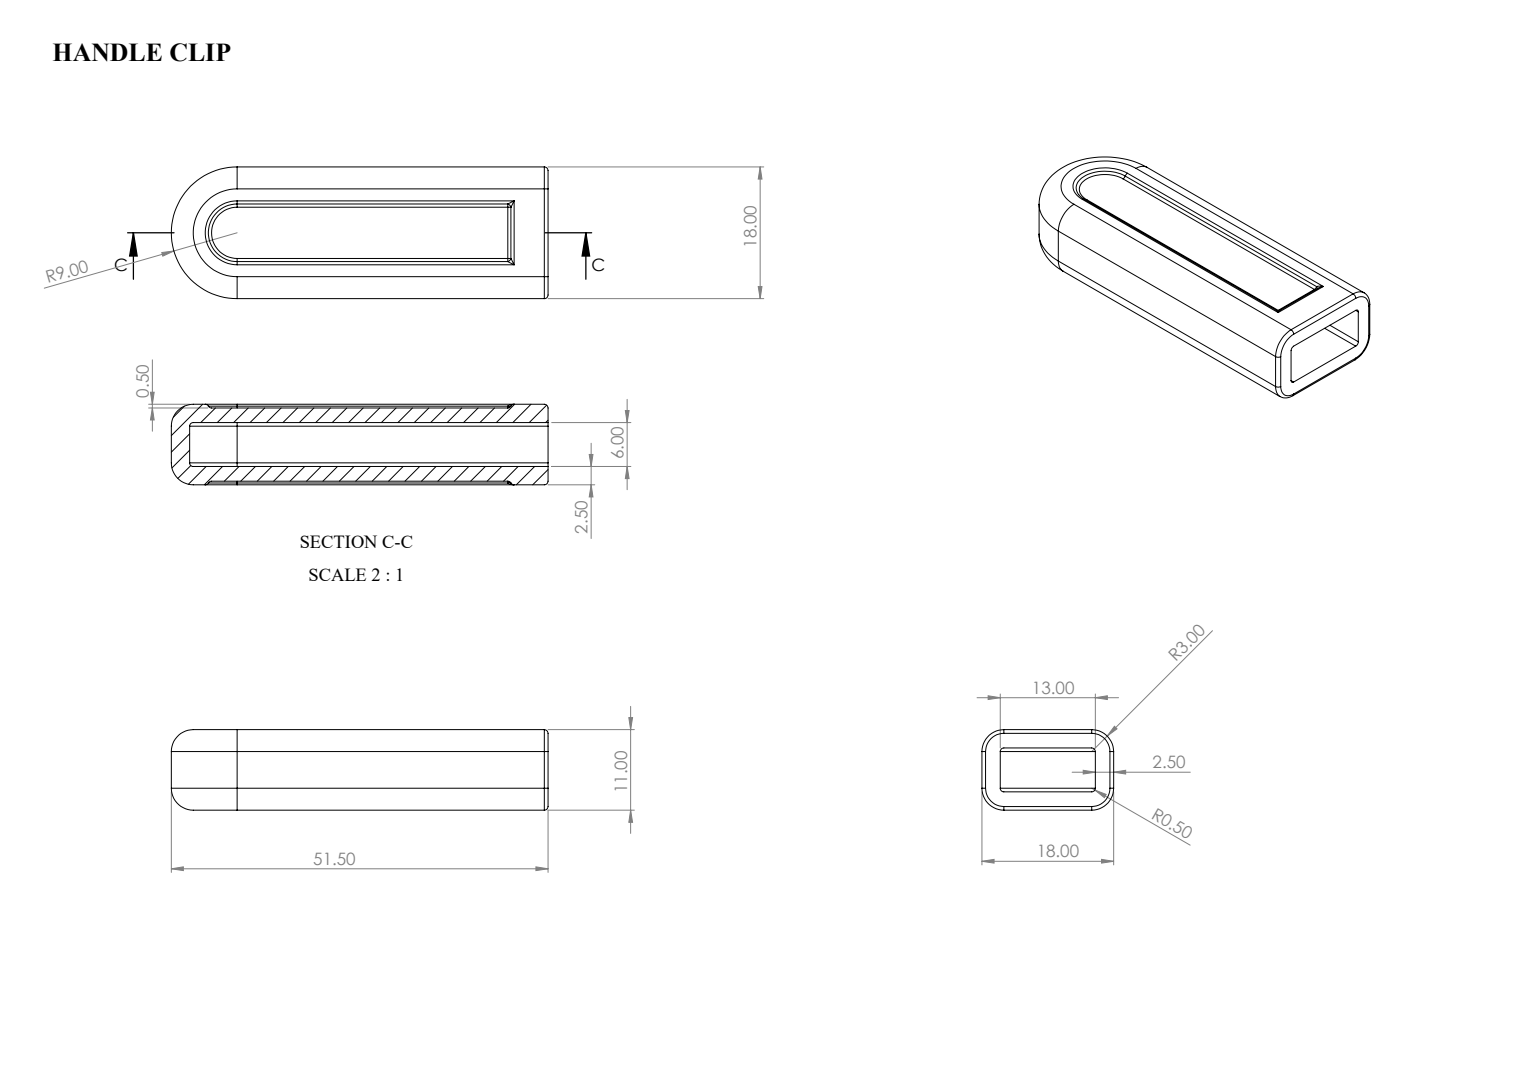
ISO-10303-21;
HEADER;
FILE_DESCRIPTION (('STEP AP214'),
    '1' );
FILE_NAME ('Handle Clip.step',
    '2026-10-06T08:09:25',
    ( '' ),
    ( '' ),
    'SwSTEP 2.0',
    'SolidWorks 2021',
    '' );
FILE_SCHEMA (( 'AUTOMOTIVE_DESIGN' ));
ENDSEC;

DATA;
#11=DIRECTION ( 'NONE',  ( 1.000000000000000000, -4.190823558986610327E-31, 1.733449886265890494E-32 ) ) ;
#13=CARTESIAN_POINT ( 'NONE',  ( 2.775557561562891351E-14, 10.75000000000000000, -10.43301270189220276 ) ) ;
#17=CARTESIAN_POINT ( 'NONE',  ( 2.775557561562891351E-14, 11.00000000000000000, -6.499999999999950262 ) ) ;
#23=CARTESIAN_POINT ( 'NONE',  ( 2.775557561562891351E-14, 8.000000000000003553, -6.499999999999950262 ) ) ;
#34=ORIENTED_EDGE ( 'NONE', *, *, #10798, .T. ) ;
#55=EDGE_CURVE ( 'NONE', #3237, #11583, #13792, .T. ) ;
#60=ORIENTED_EDGE ( 'NONE', *, *, #16971, .F. ) ;
#90=CIRCLE ( 'NONE', #20736, 0.5000000000000004441 ) ;
#104=CARTESIAN_POINT ( 'NONE',  ( 37.00000000000030553, 10.74999999999998579, -10.43301270189227559 ) ) ;
#180=VERTEX_POINT ( 'NONE', #3214 ) ;
#181=ORIENTED_EDGE ( 'NONE', *, *, #18463, .F. ) ;
#221=CARTESIAN_POINT ( 'NONE',  ( 37.36637401601599606, 0.3137297356303613283, -10.36637401601559105 ) ) ;
#222=ADVANCED_FACE ( 'NONE', ( #21089 ), #12579, .F. ) ;
#254=CARTESIAN_POINT ( 'NONE',  ( 37.09721192197999073, 0.1772999597157984553, -2.518381337117822305 ) ) ;
#264=DIRECTION ( 'NONE',  ( 1.000000000000000000, -4.190823558986610327E-31, 1.733449886265890494E-32 ) ) ;
#279=CIRCLE ( 'NONE', #13429, 0.5000000000000022204 ) ;
#288=LINE ( 'NONE', #14177, #16241 ) ;
#290=VECTOR ( 'NONE', #21577, 1000.000000000000000 ) ;
#337=ADVANCED_FACE ( 'NONE', ( #3665 ), #4392, .F. ) ;
#370=EDGE_CURVE ( 'NONE', #12160, #6309, #12209, .T. ) ;
#393=EDGE_CURVE ( 'NONE', #22556, #13205, #17081, .T. ) ;
#423=EDGE_LOOP ( 'NONE', ( #4977, #10308, #16171, #6608 ) ) ;
#435=DIRECTION ( 'NONE',  ( -1.000000000000000000, 4.190823558986610327E-31, -1.733449886265890494E-32 ) ) ;
#444=VECTOR ( 'NONE', #613, 1000.000000000000000 ) ;
#448=EDGE_CURVE ( 'NONE', #12541, #7709, #4224, .T. ) ;
#452=CARTESIAN_POINT ( 'NONE',  ( 37.00000000000006395, 10.75000000000000000, -10.43301270189220276 ) ) ;
#471=CARTESIAN_POINT ( 'NONE',  ( 42.50000000000014921, 2.999999999999999112, -14.99999999999998579 ) ) ;
#473=ADVANCED_FACE ( 'NONE', ( #13534 ), #11758, .F. ) ;
#478=AXIS2_PLACEMENT_3D ( 'NONE', #12426, #1725, #23034 ) ;
#481=ORIENTED_EDGE ( 'NONE', *, *, #4021, .F. ) ;
#485=PLANE ( 'NONE',  #3877 ) ;
#513=ORIENTED_EDGE ( 'NONE', *, *, #17633, .T. ) ;
#518=ORIENTED_EDGE ( 'NONE', *, *, #5953, .T. ) ;
#534=DIRECTION ( 'NONE',  ( 1.000000000000000000, -4.190823558986610327E-31, 1.733449886265890494E-32 ) ) ;
#539=CARTESIAN_POINT ( 'NONE',  ( 37.46001462128848658, 10.83019807384524391, -2.539985378711986819 ) ) ;
#567=EDGE_CURVE ( 'NONE', #9447, #4397, #14113, .T. ) ;
#591=EDGE_CURVE ( 'NONE', #7197, #2718, #10576, .T. ) ;
#594=EDGE_CURVE ( 'NONE', #12892, #3237, #956, .T. ) ;
#599=EDGE_LOOP ( 'NONE', ( #7573, #20564, #19035, #15482 ) ) ;
#602=CARTESIAN_POINT ( 'NONE',  ( 37.35148779274769026, 0.3618892054749011655, -2.648512207251555228 ) ) ;
#613=DIRECTION ( 'NONE',  ( 1.000000000000000000, -4.437342591868175641E-31, 3.330669073875457788E-16 ) ) ;
#614=DIRECTION ( 'NONE',  ( 0.000000000000000000, 0.000000000000000000, 1.000000000000000000 ) ) ;
#621=FACE_OUTER_BOUND ( 'NONE', #4835, .T. ) ;
#633=ORIENTED_EDGE ( 'NONE', *, *, #21096, .F. ) ;
#637=DIRECTION ( 'NONE',  ( 3.330669073875457788E-16, 0.000000000000000000, -1.000000000000000000 ) ) ;
#640=DIRECTION ( 'NONE',  ( -0.000000000000000000, 1.000000000000000000, 4.190823558986611203E-31 ) ) ;
#643=EDGE_CURVE ( 'NONE', #2718, #1098, #1705, .T. ) ;
#649=CARTESIAN_POINT ( 'NONE',  ( 2.775557561562891351E-14, 8.499999999999984013, -0.4999999999999865663 ) ) ;
#663=ORIENTED_EDGE ( 'NONE', *, *, #7766, .F. ) ;
#698=CARTESIAN_POINT ( 'NONE',  ( 2.775557561562891351E-14, 8.499999999999984013, -0.4999999999999865663 ) ) ;
#732=CARTESIAN_POINT ( 'NONE',  ( 2.775557561562891351E-14, 2.999999999999992450, -0.4999999999999865663 ) ) ;
#842=AXIS2_PLACEMENT_3D ( 'NONE', #19098, #1117, #4968 ) ;
#862=ORIENTED_EDGE ( 'NONE', *, *, #5242, .F. ) ;
#863=TOROIDAL_SURFACE ( 'NONE', #8360, 4.366025403784441039, 0.5000000000000000000 ) ;
#871=CARTESIAN_POINT ( 'NONE',  ( 37.43301270189236618, 10.75000000000000000, -2.999999999999988898 ) ) ;
#872=AXIS2_PLACEMENT_3D ( 'NONE', #21088, #8383, #18976 ) ;
#892=ORIENTED_EDGE ( 'NONE', *, *, #22327, .T. ) ;
#895=ORIENTED_EDGE ( 'NONE', *, *, #16706, .T. ) ;
#896=EDGE_CURVE ( 'NONE', #16369, #9334, #7402, .T. ) ;
#905=DIRECTION ( 'NONE',  ( 4.190823558986625216E-31, -1.000000000000000000, 4.190823558986625216E-31 ) ) ;
#906=VECTOR ( 'NONE', #1561, 1000.000000000000000 ) ;
#909=CIRCLE ( 'NONE', #17036, 0.5000000000000022204 ) ;
#918=CARTESIAN_POINT ( 'NONE',  ( 37.57823792062865209, 0.08880391167987312928, -10.29045043747235333 ) ) ;
#956=CIRCLE ( 'NONE', #20106, 3.933012701892234730 ) ;
#966=FACE_OUTER_BOUND ( 'NONE', #6498, .T. ) ;
#971=DIRECTION ( 'NONE',  ( 0.000000000000000000, 0.000000000000000000, 1.000000000000000000 ) ) ;
#977=ORIENTED_EDGE ( 'NONE', *, *, #23196, .F. ) ;
#980=ORIENTED_EDGE ( 'NONE', *, *, #4067, .T. ) ;
#999=CARTESIAN_POINT ( 'NONE',  ( 37.00000000000011369, 10.49999999999999822, -10.00000000000000888 ) ) ;
#1005=ORIENTED_EDGE ( 'NONE', *, *, #896, .T. ) ;
#1019=FACE_OUTER_BOUND ( 'NONE', #2701, .T. ) ;
#1038=ORIENTED_EDGE ( 'NONE', *, *, #6940, .T. ) ;
#1043=DIRECTION ( 'NONE',  ( -4.190823558986626092E-31, 1.000000000000000000, 4.190823558986610327E-31 ) ) ;
#1069=ADVANCED_FACE ( 'NONE', ( #22690 ), #22337, .T. ) ;
#1071=EDGE_CURVE ( 'NONE', #22556, #2883, #22565, .T. ) ;
#1076=CARTESIAN_POINT ( 'NONE',  ( 37.00000000000011369, 11.00000000000000000, -6.499999999999950262 ) ) ;
#1098=VERTEX_POINT ( 'NONE', #13743 ) ;
#1117=DIRECTION ( 'NONE',  ( -1.000000000000000000, 4.190823558986610327E-31, -1.733449886265890494E-32 ) ) ;
#1149=SHAPE_REPRESENTATION_RELATIONSHIP ( 'NONE' , 'NONE' ,  #1164, #3571 ) ;
#1154=ORIENTED_EDGE ( 'NONE', *, *, #9823, .F. ) ;
#1164=SHAPE_REPRESENTATION ( 'Handle Clip', ( #22115 ), #13848 ) ;
#1185=CARTESIAN_POINT ( 'NONE',  ( 2.775557561562891351E-14, 0.5000000000000004441, -3.000000000000002665 ) ) ;
#1188=SPHERICAL_SURFACE ( 'NONE', #17017, 0.5000000000000000000 ) ;
#1193=CARTESIAN_POINT ( 'NONE',  ( 37.43301270189239460, 0.2500000000000002220, -9.999999999999953815 ) ) ;
#1228=CIRCLE ( 'NONE', #14361, 0.5000000000000004441 ) ;
#1229=DIRECTION ( 'NONE',  ( -0.000000000000000000, 1.000000000000000000, 4.190823558986611203E-31 ) ) ;
#1236=ORIENTED_EDGE ( 'NONE', *, *, #23063, .T. ) ;
#1238=ORIENTED_EDGE ( 'NONE', *, *, #15588, .F. ) ;
#1256=AXIS2_PLACEMENT_3D ( 'NONE', #7873, #3869, #9180 ) ;
#1287=CYLINDRICAL_SURFACE ( 'NONE', #4701, 0.5000000000000017764 ) ;
#1302=DIRECTION ( 'NONE',  ( -4.190823558986625216E-31, 1.000000000000000000, -4.190823558986625216E-31 ) ) ;
#1322=ORIENTED_EDGE ( 'NONE', *, *, #5382, .T. ) ;
#1341=CARTESIAN_POINT ( 'NONE',  ( 37.00000000000017053, 0.2500000000000002220, -10.43301270189217433 ) ) ;
#1361=AXIS2_PLACEMENT_3D ( 'NONE', #12480, #2122, #5209 ) ;
#1365=DIRECTION ( 'NONE',  ( -1.000000000000000000, 4.190823558986610327E-31, -1.733449886265890494E-32 ) ) ;
#1366=STYLED_ITEM ( 'NONE', ( #22113 ), #21090 ) ;
#1373=DIRECTION ( 'NONE',  ( 0.000000000000000000, 9.769962616701412266E-15, 1.000000000000000000 ) ) ;
#1379=FILL_AREA_STYLE ('',( #17353 ) ) ;
#1390=CARTESIAN_POINT ( 'NONE',  ( 42.00000000000020606, 0.4999999999999865663, -0.4999999999999449329 ) ) ;
#1394=DIRECTION ( 'NONE',  ( 3.330669073875454830E-16, 0.000000000000000000, -1.000000000000000000 ) ) ;
#1416=CARTESIAN_POINT ( 'NONE',  ( 2.775557561562891351E-14, 11.00000000000000000, -9.999999999999968026 ) ) ;
#1455=EDGE_CURVE ( 'NONE', #5339, #2694, #13565, .T. ) ;
#1462=CIRCLE ( 'NONE', #22131, 4.366025403784456138 ) ;
#1467=EDGE_CURVE ( 'NONE', #15040, #9447, #5099, .T. ) ;
#1476=DIRECTION ( 'NONE',  ( 0.000000000000000000, 0.000000000000000000, -1.000000000000000000 ) ) ;
#1479=DIRECTION ( 'NONE',  ( -1.000000000000000000, 0.000000000000000000, 0.000000000000000000 ) ) ;
#1481=DIRECTION ( 'NONE',  ( 0.000000000000000000, -4.190823558986610327E-31, 1.000000000000000000 ) ) ;
#1526=FACE_OUTER_BOUND ( 'NONE', #8749, .T. ) ;
#1536=CARTESIAN_POINT ( 'NONE',  ( 37.18301270189237329, 10.90849364905388619, -2.475480947161653233 ) ) ;
#1556=DIRECTION ( 'NONE',  ( 0.000000000000000000, 0.000000000000000000, 1.000000000000000000 ) ) ;
#1559=DIRECTION ( 'NONE',  ( -4.190823558986625216E-31, 1.000000000000000000, -4.190823558986625216E-31 ) ) ;
#1561=DIRECTION ( 'NONE',  ( -4.190823558986625216E-31, 1.000000000000000000, -4.190823558986625216E-31 ) ) ;
#1562=CYLINDRICAL_SURFACE ( 'NONE', #18135, 0.5000000000000022204 ) ;
#1581=ORIENTED_EDGE ( 'NONE', *, *, #20471, .T. ) ;
#1582=CARTESIAN_POINT ( 'NONE',  ( 42.00000000000012079, 2.999999999999999112, -12.49999999999999645 ) ) ;
#1591=ADVANCED_FACE ( 'NONE', ( #21452 ), #10724, .T. ) ;
#1605=ADVANCED_FACE ( 'NONE', ( #9075 ), #23102, .F. ) ;
#1624=CARTESIAN_POINT ( 'NONE',  ( 37.73505106183036162, 10.99999999999229061, -10.73505106183359104 ) ) ;
#1630=LINE ( 'NONE', #8813, #3292 ) ;
#1646=DIRECTION ( 'NONE',  ( 4.190823558986625216E-31, -1.000000000000000000, 4.190823558986625216E-31 ) ) ;
#1656=DIRECTION ( 'NONE',  ( -1.000000000000000000, 4.190823558986610327E-31, -1.733449886265890494E-32 ) ) ;
#1658=CARTESIAN_POINT ( 'NONE',  ( 37.68301270189240171, 11.00000000000000533, -2.499999999999975575 ) ) ;
#1669=VERTEX_POINT ( 'NONE', #11524 ) ;
#1705=CIRCLE ( 'NONE', #16346, 2.500000000000009326 ) ;
#1725=DIRECTION ( 'NONE',  ( 4.392831559381931789E-32, 2.168404344970994323E-16, 1.000000000000000000 ) ) ;
#1727=FACE_OUTER_BOUND ( 'NONE', #17848, .T. ) ;
#1734=CARTESIAN_POINT ( 'NONE',  ( 37.77870956205628516, 11.00000000000000000, -10.69139372032722335 ) ) ;
#1746=ORIENTED_EDGE ( 'NONE', *, *, #17889, .F. ) ;
#1759=CARTESIAN_POINT ( 'NONE',  ( 2.775557561562891351E-14, 8.500000000000003553, -6.499999999999950262 ) ) ;
#1764=DIRECTION ( 'NONE',  ( 1.000000000000000000, -4.190823558986610327E-31, 1.733449886265890494E-32 ) ) ;
#1823=CARTESIAN_POINT ( 'NONE',  ( 2.775557561562891351E-14, 11.00000000000000000, -12.50000000000001066 ) ) ;
#1836=CARTESIAN_POINT ( 'NONE',  ( 42.50000000000014921, 5.500000000000001776, 2.000000000000071054 ) ) ;
#1890=DIRECTION ( 'NONE',  ( -1.000000000000000000, 4.190823558986610327E-31, -1.733449886265890494E-32 ) ) ;
#1926=CIRCLE ( 'NONE', #17697, 3.000000000000011546 ) ;
#1960=CARTESIAN_POINT ( 'NONE',  ( 37.45482484129320966, 0.2122202663360098496, -10.04362427881557274 ) ) ;
#1965=EDGE_LOOP ( 'NONE', ( #1982, #10746, #15822, #4725 ) ) ;
#1966=EDGE_CURVE ( 'NONE', #3408, #6309, #5169, .T. ) ;
#1982=ORIENTED_EDGE ( 'NONE', *, *, #448, .F. ) ;
#1985=LINE ( 'NONE', #7524, #10565 ) ;
#2000=ORIENTED_EDGE ( 'NONE', *, *, #370, .T. ) ;
#2003=ORIENTED_EDGE ( 'NONE', *, *, #17889, .T. ) ;
#2006=EDGE_CURVE ( 'NONE', #13205, #15190, #3678, .T. ) ;
#2009=CIRCLE ( 'NONE', #18541, 3.933012701892234730 ) ;
#2016=CARTESIAN_POINT ( 'NONE',  ( 2.775557561562891351E-14, 10.49999999999999822, -9.999999999999968026 ) ) ;
#2020=CARTESIAN_POINT ( 'NONE',  ( 42.50000000000020606, 2.499999999999998668, -13.00000000000002487 ) ) ;
#2030=ORIENTED_EDGE ( 'NONE', *, *, #21313, .F. ) ;
#2045=DIRECTION ( 'NONE',  ( -1.000000000000000000, 4.437342591868175641E-31, -3.330669073875457788E-16 ) ) ;
#2108=DIRECTION ( 'NONE',  ( 1.000000000000000000, -4.190823558986610327E-31, 1.733449886265890494E-32 ) ) ;
#2112=SHAPE_DEFINITION_REPRESENTATION ( #15484, #1164 ) ;
#2117=ORIENTED_EDGE ( 'NONE', *, *, #5918, .F. ) ;
#2122=DIRECTION ( 'NONE',  ( 1.733449886265891589E-32, -4.190823558986610327E-31, 1.000000000000000000 ) ) ;
#2130=LINE ( 'NONE', #16478, #444 ) ;
#2141=AXIS2_PLACEMENT_3D ( 'NONE', #5036, #12437, #3627 ) ;
#2143=ORIENTED_EDGE ( 'NONE', *, *, #22541, .T. ) ;
#2148=CIRCLE ( 'NONE', #6298, 0.5000000000000012212 ) ;
#2162=DIRECTION ( 'NONE',  ( 0.000000000000000000, 0.000000000000000000, -1.000000000000000000 ) ) ;
#2181=ORIENTED_EDGE ( 'NONE', *, *, #14586, .T. ) ;
#2182=AXIS2_PLACEMENT_3D ( 'NONE', #11996, #13664, #17057 ) ;
#2187=CARTESIAN_POINT ( 'NONE',  ( 2.775557561562891351E-14, 2.999999999999999112, -12.50000000000001066 ) ) ;
#2193=CARTESIAN_POINT ( 'NONE',  ( 5.551115123125782702E-14, 3.000000000000027089, 2.500000000000071498 ) ) ;
#2247=ORIENTED_EDGE ( 'NONE', *, *, #14877, .T. ) ;
#2355=CARTESIAN_POINT ( 'NONE',  ( 37.29045043747246524, 0.08880391167994924895, -2.421762079371568621 ) ) ;
#2357=VERTEX_POINT ( 'NONE', #12661 ) ;
#2365=CARTESIAN_POINT ( 'NONE',  ( 42.00000000000014921, 10.49999999999999822, -12.50000000000005329 ) ) ;
#2406=CIRCLE ( 'NONE', #14045, 6.500000000000023981 ) ;
#2436=AXIS2_PLACEMENT_3D ( 'NONE', #5086, #19320, #17907 ) ;
#2449=VECTOR ( 'NONE', #22347, 1000.000000000000000 ) ;
#2453=CARTESIAN_POINT ( 'NONE',  ( 42.00000000000020606, -1.387778780781445676E-14, -0.4999999999999449329 ) ) ;
#2463=EDGE_CURVE ( 'NONE', #3085, #7197, #14612, .T. ) ;
#2469=LINE ( 'NONE', #6127, #2740 ) ;
#2524=ORIENTED_EDGE ( 'NONE', *, *, #1467, .T. ) ;
#2536=LINE ( 'NONE', #7952, #7258 ) ;
#2541=VECTOR ( 'NONE', #5687, 1000.000000000000000 ) ;
#2546=CARTESIAN_POINT ( 'NONE',  ( 37.73505106183116453, 7.752354164078167471E-12, -10.73505106183309543 ) ) ;
#2547=VECTOR ( 'NONE', #4832, 1000.000000000000000 ) ;
#2570=DIRECTION ( 'NONE',  ( 1.000000000000000000, -4.190823558986610327E-31, 1.733449886265890494E-32 ) ) ;
#2575=DIRECTION ( 'NONE',  ( 4.190823558986625216E-31, -1.000000000000000000, 4.190823558986625216E-31 ) ) ;
#2586=CARTESIAN_POINT ( 'NONE',  ( 2.775557561562891351E-14, 2.499999999999998668, -6.499999999999950262 ) ) ;
#2589=ORIENTED_EDGE ( 'NONE', *, *, #13484, .F. ) ;
#2615=( BOUNDED_CURVE ( )  B_SPLINE_CURVE ( 3, ( #11377, #12923, #10910, #452 ),
 .UNSPECIFIED., .F., .F. ) 
 B_SPLINE_CURVE_WITH_KNOTS ( ( 4, 4 ),
 ( 1.570796326794896558, 2.617993877991555252 ),
 .UNSPECIFIED. ) 
 CURVE ( )  GEOMETRIC_REPRESENTATION_ITEM ( )  RATIONAL_B_SPLINE_CURVE ( ( 1.000000000000000000, 0.9106836025229487763, 0.9106836025229487763, 1.000000000000000000 ) ) 
 REPRESENTATION_ITEM ( '' )  );
#2625=AXIS2_PLACEMENT_3D ( 'NONE', #11795, #8154, #20750 ) ;
#2631=CARTESIAN_POINT ( 'NONE',  ( 42.00000000000014921, 2.999999999999999112, -15.00000000000001421 ) ) ;
#2656=AXIS2_PLACEMENT_3D ( 'NONE', #6369, #13310, #14944 ) ;
#2681=CARTESIAN_POINT ( 'NONE',  ( 2.775557561562891351E-14, 8.500000000000003553, -6.499999999999950262 ) ) ;
#2693=ORIENTED_EDGE ( 'NONE', *, *, #12821, .F. ) ;
#2694=VERTEX_POINT ( 'NONE', #20789 ) ;
#2696=CIRCLE ( 'NONE', #9847, 0.5000000000000004441 ) ;
#2701=EDGE_LOOP ( 'NONE', ( #12986, #7252, #2247, #12420 ) ) ;
#2708=CYLINDRICAL_SURFACE ( 'NONE', #11715, 9.000000000000031974 ) ;
#2714=DIRECTION ( 'NONE',  ( 0.000000000000000000, 0.000000000000000000, 1.000000000000000000 ) ) ;
#2718=VERTEX_POINT ( 'NONE', #22660 ) ;
#2722=ORIENTED_EDGE ( 'NONE', *, *, #7766, .T. ) ;
#2740=VECTOR ( 'NONE', #16468, 1000.000000000000000 ) ;
#2758=AXIS2_PLACEMENT_3D ( 'NONE', #16955, #13884, #15520 ) ;
#2805=DIRECTION ( 'NONE',  ( -4.190823558986626092E-31, 1.000000000000000000, 4.190823558986610327E-31 ) ) ;
#2807=( BOUNDED_CURVE ( )  B_SPLINE_CURVE ( 3, ( #5658, #9761, #18585, #18238 ),
 .UNSPECIFIED., .F., .T. ) 
 B_SPLINE_CURVE_WITH_KNOTS ( ( 4, 4 ),
 ( 3.665191429188058070, 4.712388980384689674 ),
 .UNSPECIFIED. ) 
 CURVE ( )  GEOMETRIC_REPRESENTATION_ITEM ( )  RATIONAL_B_SPLINE_CURVE ( ( 1.000000000000000000, 0.9106836025229534393, 0.9106836025229534393, 1.000000000000000000 ) ) 
 REPRESENTATION_ITEM ( '' )  );
#2841=FACE_OUTER_BOUND ( 'NONE', #18394, .T. ) ;
#2843=CARTESIAN_POINT ( 'NONE',  ( 2.775557561562891351E-14, 2.499999999999998668, -0.4999999999999865663 ) ) ;
#2856=DIRECTION ( 'NONE',  ( 1.000000000000000000, -4.437342591868175641E-31, 3.330669073875457788E-16 ) ) ;
#2866=MECHANICAL_DESIGN_GEOMETRIC_PRESENTATION_REPRESENTATION('',(#1366),#11878);
#2875=EDGE_LOOP ( 'NONE', ( #16462, #11920, #15706, #980 ) ) ;
#2883=VERTEX_POINT ( 'NONE', #17832 ) ;
#2885=CARTESIAN_POINT ( 'NONE',  ( 2.775557561562891351E-14, 10.49999999999998579, -2.133974596215532316 ) ) ;
#2908=ORIENTED_EDGE ( 'NONE', *, *, #567, .F. ) ;
#2963=DIRECTION ( 'NONE',  ( 0.000000000000000000, 0.000000000000000000, 1.000000000000000000 ) ) ;
#2975=CARTESIAN_POINT ( 'NONE',  ( 2.775557561562891351E-14, 0.2500000000000106581, -10.43301270189220276 ) ) ;
#3013=DIRECTION ( 'NONE',  ( -1.733449886265891589E-32, 4.190823558986610327E-31, -1.000000000000000000 ) ) ;
#3027=ORIENTED_EDGE ( 'NONE', *, *, #4619, .F. ) ;
#3028=ORIENTED_EDGE ( 'NONE', *, *, #22353, .F. ) ;
#3042=DIRECTION ( 'NONE',  ( 0.000000000000000000, 0.000000000000000000, -1.000000000000000000 ) ) ;
#3051=ORIENTED_EDGE ( 'NONE', *, *, #17748, .F. ) ;
#3056=ORIENTED_EDGE ( 'NONE', *, *, #15395, .T. ) ;
#3059=DIRECTION ( 'NONE',  ( 1.000000000000000000, -4.190823558986610327E-31, 1.733449886265890494E-32 ) ) ;
#3072=CYLINDRICAL_SURFACE ( 'NONE', #2182, 0.5000000000000017764 ) ;
#3084=ORIENTED_EDGE ( 'NONE', *, *, #6771, .F. ) ;
#3085=VERTEX_POINT ( 'NONE', #15328 ) ;
#3088=ORIENTED_EDGE ( 'NONE', *, *, #9695, .F. ) ;
#3145=SURFACE_STYLE_FILL_AREA ( #1379 ) ;
#3147=DIRECTION ( 'NONE',  ( -1.000000000000000000, 4.190823558986610327E-31, -1.733449886265890494E-32 ) ) ;
#3167=DIRECTION ( 'NONE',  ( 1.000000000000000000, -4.437342591868175641E-31, 3.330669073875457788E-16 ) ) ;
#3182=ADVANCED_FACE ( 'NONE', ( #3753 ), #19067, .T. ) ;
#3189=FACE_OUTER_BOUND ( 'NONE', #8380, .T. ) ;
#3214=CARTESIAN_POINT ( 'NONE',  ( 2.775557561562891351E-14, 8.500000000000003553, -12.50000000000001066 ) ) ;
#3216=CARTESIAN_POINT ( 'NONE',  ( 37.00000000000014211, 0.000000000000000000, -9.999999999999980460 ) ) ;
#3219=EDGE_CURVE ( 'NONE', #13762, #18075, #2148, .T. ) ;
#3237=VERTEX_POINT ( 'NONE', #9412 ) ;
#3252=CARTESIAN_POINT ( 'NONE',  ( 42.50000000000012079, 10.49999999999999822, -0.4999999999999865663 ) ) ;
#3254=CYLINDRICAL_SURFACE ( 'NONE', #9503, 0.5000000000000004441 ) ;
#3267=AXIS2_PLACEMENT_3D ( 'NONE', #4885, #10303, #21135 ) ;
#3292=VECTOR ( 'NONE', #8690, 1000.000000000000000 ) ;
#3303=VECTOR ( 'NONE', #8021, 1000.000000000000000 ) ;
#3311=VECTOR ( 'NONE', #7956, 1000.000000000000000 ) ;
#3359=AXIS2_PLACEMENT_3D ( 'NONE', #4417, #20795, #1373 ) ;
#3377=DIRECTION ( 'NONE',  ( 1.000000000000000000, 1.492474417944841737E-16, 3.842941406090992613E-32 ) ) ;
#3378=DIRECTION ( 'NONE',  ( -1.733449886265890494E-32, -4.190823558986611203E-31, 1.000000000000000000 ) ) ;
#3388=EDGE_LOOP ( 'NONE', ( #19454, #20353, #18890 ) ) ;
#3390=LINE ( 'NONE', #17722, #12919 ) ;
#3399=CARTESIAN_POINT ( 'NONE',  ( 0.000000000000000000, 11.00000000000000000, -10.86602540378443749 ) ) ;
#3401=CARTESIAN_POINT ( 'NONE',  ( 37.46001462128847947, 10.83019807384524036, -10.46001462128798210 ) ) ;
#3408=VERTEX_POINT ( 'NONE', #19047 ) ;
#3413=ADVANCED_FACE ( 'NONE', ( #11862 ), #11529, .T. ) ;
#3417=ORIENTED_EDGE ( 'NONE', *, *, #2463, .F. ) ;
#3426=CARTESIAN_POINT ( 'NONE',  ( 2.775557561562891351E-14, 2.999999999999999112, -6.499999999999950262 ) ) ;
#3461=ORIENTED_EDGE ( 'NONE', *, *, #15395, .F. ) ;
#3481=EDGE_CURVE ( 'NONE', #11583, #22878, #279, .T. ) ;
#3488=AXIS2_PLACEMENT_3D ( 'NONE', #3929, #18287, #2162 ) ;
#3489=CIRCLE ( 'NONE', #12491, 3.500000000000013323 ) ;
#3510=CARTESIAN_POINT ( 'NONE',  ( 37.69160037009659447, 10.97664592903645087, -10.51717533640882962 ) ) ;
#3518=ADVANCED_FACE ( 'NONE', ( #18932 ), #21046, .T. ) ;
#3529=APPLICATION_CONTEXT ( 'automotive_design' ) ;
#3536=CARTESIAN_POINT ( 'NONE',  ( 2.775557561562891351E-14, 2.999999999999999112, -12.50000000000001066 ) ) ;
#3543=FACE_OUTER_BOUND ( 'NONE', #11206, .T. ) ;
#3568=LINE ( 'NONE', #7214, #5792 ) ;
#3571=ADVANCED_BREP_SHAPE_REPRESENTATION ( '', ( #21090, #22115 ), #13848 ) ;
#3589=PLANE ( 'NONE',  #2758 ) ;
#3593=CARTESIAN_POINT ( 'NONE',  ( 2.775557561562891351E-14, 0.5000000000000004441, -2.133974596215532316 ) ) ;
#3598=FACE_OUTER_BOUND ( 'NONE', #9574, .T. ) ;
#3622=CARTESIAN_POINT ( 'NONE',  ( 37.69139372032788771, 10.99999999999996625, -10.77870956205603648 ) ) ;
#3623=ADVANCED_FACE ( 'NONE', ( #21741 ), #11747, .F. ) ;
#3627=DIRECTION ( 'NONE',  ( -1.000000000000000000, 0.000000000000000000, 0.000000000000000000 ) ) ;
#3646=EDGE_CURVE ( 'NONE', #15424, #18871, #5626, .T. ) ;
#3650=CARTESIAN_POINT ( 'NONE',  ( 42.00000000000020606, 8.000000000000003553, -0.4999999999999449329 ) ) ;
#3656=AXIS2_PLACEMENT_3D ( 'NONE', #18665, #6086, #9736 ) ;
#3665=FACE_OUTER_BOUND ( 'NONE', #8208, .T. ) ;
#3677=CARTESIAN_POINT ( 'NONE',  ( 2.775557561562891351E-14, 5.500000000000001776, -15.49999999999998579 ) ) ;
#3678=CIRCLE ( 'NONE', #19073, 9.000000000000031974 ) ;
#3687=EDGE_LOOP ( 'NONE', ( #6041, #1746, #4892, #16938 ) ) ;
#3696=CIRCLE ( 'NONE', #16820, 6.000000000000023093 ) ;
#3753=FACE_OUTER_BOUND ( 'NONE', #18820, .T. ) ;
#3773=AXIS2_PLACEMENT_3D ( 'NONE', #17, #18005, #7303 ) ;
#3786=EDGE_CURVE ( 'NONE', #12541, #21020, #15305, .T. ) ;
#3816=FACE_OUTER_BOUND ( 'NONE', #8321, .T. ) ;
#3824=CIRCLE ( 'NONE', #14357, 3.000000000000011102 ) ;
#3837=CARTESIAN_POINT ( 'NONE',  ( 37.22062532321636752, 10.88440674090235305, -10.54332536350028882 ) ) ;
#3849=EDGE_LOOP ( 'NONE', ( #17324, #22882, #12393 ) ) ;
#3861=ORIENTED_EDGE ( 'NONE', *, *, #9614, .T. ) ;
#3869=DIRECTION ( 'NONE',  ( 1.000000000000000000, -4.190823558986610327E-31, 1.733449886265890494E-32 ) ) ;
#3874=VECTOR ( 'NONE', #16784, 1000.000000000000000 ) ;
#3877=AXIS2_PLACEMENT_3D ( 'NONE', #14829, #18472, #9539 ) ;
#3924=EDGE_CURVE ( 'NONE', #16351, #1669, #7845, .T. ) ;
#3929=CARTESIAN_POINT ( 'NONE',  ( 2.775557561562891351E-14, 7.999999999999983125, -0.4999999999999865663 ) ) ;
#3933=EDGE_CURVE ( 'NONE', #9334, #16286, #1462, .T. ) ;
#3937=CARTESIAN_POINT ( 'NONE',  ( 37.54332536350037230, 10.88440674090231752, -2.779374676783941567 ) ) ;
#3943=VERTEX_POINT ( 'NONE', #1823 ) ;
#3952=CYLINDRICAL_SURFACE ( 'NONE', #6841, 0.5000000000000022204 ) ;
#3962=APPLICATION_CONTEXT ( 'automotive_design' ) ;
#3983=VECTOR ( 'NONE', #17623, 1000.000000000000000 ) ;
#4009=VECTOR ( 'NONE', #17544, 1000.000000000000000 ) ;
#4018=CARTESIAN_POINT ( 'NONE',  ( 42.50000000000023448, 10.49999999999999822, 2.500000000000002220 ) ) ;
#4021=EDGE_CURVE ( 'NONE', #13762, #13703, #16544, .T. ) ;
#4041=DIRECTION ( 'NONE',  ( 0.000000000000000000, 0.000000000000000000, 1.000000000000000000 ) ) ;
#4067=EDGE_CURVE ( 'NONE', #3237, #9334, #11925, .T. ) ;
#4103=LINE ( 'NONE', #20114, #11373 ) ;
#4105=SURFACE_STYLE_FILL_AREA ( #11053 ) ;
#4135=ORIENTED_EDGE ( 'NONE', *, *, #15331, .F. ) ;
#4145=ORIENTED_EDGE ( 'NONE', *, *, #5242, .T. ) ;
#4158=CIRCLE ( 'NONE', #17303, 0.5000000000000022204 ) ;
#4166=ORIENTED_EDGE ( 'NONE', *, *, #16706, .F. ) ;
#4189=ORIENTED_EDGE ( 'NONE', *, *, #5953, .F. ) ;
#4193=ORIENTED_EDGE ( 'NONE', *, *, #11651, .T. ) ;
#4195=DIRECTION ( 'NONE',  ( -1.733449886265890494E-32, 7.264582621685754939E-63, 1.000000000000000000 ) ) ;
#4212=SURFACE_SIDE_STYLE ('',( #4105 ) ) ;
#4221=ORIENTED_EDGE ( 'NONE', *, *, #20349, .T. ) ;
#4224=LINE ( 'NONE', #1185, #22748 ) ;
#4231=AXIS2_PLACEMENT_3D ( 'NONE', #21434, #14004, #5301 ) ;
#4248=EDGE_LOOP ( 'NONE', ( #4166, #3417, #4430, #8421 ) ) ;
#4270=LINE ( 'NONE', #649, #10666 ) ;
#4303=CARTESIAN_POINT ( 'NONE',  ( 2.775557561562891351E-14, 2.499999999999998668, -6.499999999999950262 ) ) ;
#4326=DIRECTION ( 'NONE',  ( 0.4472135954999523766, 0.7745966692414836263, -0.4472135954999632568 ) ) ;
#4331=ADVANCED_FACE ( 'NONE', ( #15332 ), #22632, .F. ) ;
#4338=EDGE_CURVE ( 'NONE', #7712, #12541, #22834, .T. ) ;
#4351=DIRECTION ( 'NONE',  ( -1.756300210255732376E-61, 4.190823558986625216E-31, 1.000000000000000000 ) ) ;
#4392=( BOUNDED_SURFACE ( )  B_SPLINE_SURFACE ( 3, 2, ( 
 ( #9071, #9308, #18368 ),
 ( #10940, #602, #16230 ),
 ( #254, #11064, #18132 ),
 ( #5788, #22007, #9195 ),
 ( #2355, #16353, #7431 ),
 ( #16469, #18249, #21789 ),
 ( #9540, #16694, #7765 ),
 ( #9425, #5672, #10837 ) ),
 .UNSPECIFIED., .F., .F., .F. ) 
 B_SPLINE_SURFACE_WITH_KNOTS ( ( 4, 2, 2, 4 ),
 ( 3, 3 ),
 ( 3.665191429188093597, 3.926990816987242283, 4.188790204786391413, 4.712388980384689674 ),
 ( 0.000000000000000000, 1.000000000000000000 ),
 .UNSPECIFIED. ) 
 GEOMETRIC_REPRESENTATION_ITEM ( )  RATIONAL_B_SPLINE_SURFACE ( (
 ( 1.000000000000000000, 0.7905694150421759270, 1.000000000000000000),
 ( 1.000000000000000000, 0.8144940154005636535, 1.000000000000000000),
 ( 1.000000000000000000, 0.8408337562111811714, 1.000000000000000000),
 ( 1.000000000000000000, 0.8912170513578138165, 1.000000000000000000),
 ( 1.000000000000000000, 0.9152160911082614092, 1.000000000000000000),
 ( 1.000000000000000000, 0.9758108578640474207, 1.000000000000000000),
 ( 1.000000000000000000, 1.000509427570048571, 1.000000000000000000),
 ( 1.000000000000000000, 1.000000000000000000, 1.000000000000000000) ) ) 
 REPRESENTATION_ITEM ( '' )  SURFACE ( )  );
#4397=VERTEX_POINT ( 'NONE', #10850 ) ;
#4398=EDGE_CURVE ( 'NONE', #7856, #9447, #5573, .T. ) ;
#4417=CARTESIAN_POINT ( 'NONE',  ( 37.00000000000014211, 0.000000000000000000, -3.000000000000002665 ) ) ;
#4424=( NAMED_UNIT ( * ) PLANE_ANGLE_UNIT ( ) SI_UNIT ( $, .RADIAN. ) );
#4430=ORIENTED_EDGE ( 'NONE', *, *, #12114, .F. ) ;
#4436=EDGE_LOOP ( 'NONE', ( #22147, #13709, #1581, #1038 ) ) ;
#4449=CARTESIAN_POINT ( 'NONE',  ( 0.000000000000000000, 2.999999999999992450, 0.000000000000000000 ) ) ;
#4476=DIRECTION ( 'NONE',  ( 4.190823558986625216E-31, -1.000000000000000000, 4.190823558986625216E-31 ) ) ;
#4490=ORIENTED_EDGE ( 'NONE', *, *, #18153, .T. ) ;
#4498=VERTEX_POINT ( 'NONE', #21687 ) ;
#4512=CARTESIAN_POINT ( 'NONE',  ( 37.52451905283846401, 0.09150635094610139186, -2.816987298107726634 ) ) ;
#4529=ORIENTED_EDGE ( 'NONE', *, *, #10067, .F. ) ;
#4532=FACE_OUTER_BOUND ( 'NONE', #4699, .T. ) ;
#4566=CARTESIAN_POINT ( 'NONE',  ( 2.775557561562891351E-14, 8.000000000000003553, -12.50000000000001066 ) ) ;
#4585=CARTESIAN_POINT ( 'NONE',  ( 2.775557561562891351E-14, 10.49999999999998579, -3.000000000000002665 ) ) ;
#4612=CARTESIAN_POINT ( 'NONE',  ( 2.775557561562891351E-14, 7.999999999999983125, -0.4999999999999865663 ) ) ;
#4618=DIRECTION ( 'NONE',  ( 1.733449886265891589E-32, -4.190823558986610327E-31, 1.000000000000000000 ) ) ;
#4619=EDGE_CURVE ( 'NONE', #5046, #9224, #14836, .T. ) ;
#4623=LINE ( 'NONE', #22983, #17035 ) ;
#4624=CARTESIAN_POINT ( 'NONE',  ( 2.775557561562891351E-14, 8.000000000000003553, -12.99999999999999822 ) ) ;
#4625=CARTESIAN_POINT ( 'NONE',  ( 37.00000000000011369, 11.00000000000000000, -10.00000000000000888 ) ) ;
#4633=AXIS2_PLACEMENT_3D ( 'NONE', #13285, #2570, #11501 ) ;
#4645=ORIENTED_EDGE ( 'NONE', *, *, #15832, .T. ) ;
#4658=AXIS2_PLACEMENT_3D ( 'NONE', #19034, #1043, #20455 ) ;
#4659=FACE_OUTER_BOUND ( 'NONE', #16373, .T. ) ;
#4666=( LENGTH_UNIT ( ) NAMED_UNIT ( * ) SI_UNIT ( .MILLI., .METRE. ) );
#4671=VERTEX_POINT ( 'NONE', #3399 ) ;
#4699=EDGE_LOOP ( 'NONE', ( #18157, #10187, #2908, #5615 ) ) ;
#4701=AXIS2_PLACEMENT_3D ( 'NONE', #8456, #15616, #11503 ) ;
#4708=CARTESIAN_POINT ( 'NONE',  ( 2.775557561562891351E-14, 2.999999999999999112, -12.50000000000001066 ) ) ;
#4712=DIRECTION ( 'NONE',  ( -1.000000000000000000, 4.437342591868175641E-31, -3.330669073875457788E-16 ) ) ;
#4725=ORIENTED_EDGE ( 'NONE', *, *, #8260, .T. ) ;
#4735=DIRECTION ( 'NONE',  ( 0.000000000000000000, 0.000000000000000000, 1.000000000000000000 ) ) ;
#4765=CARTESIAN_POINT ( 'NONE',  ( 42.50000000000014921, 0.4999999999999865663, -0.4999999999999726885 ) ) ;
#4816=AXIS2_PLACEMENT_3D ( 'NONE', #23, #21547, #15990 ) ;
#4820=ORIENTED_EDGE ( 'NONE', *, *, #3646, .F. ) ;
#4832=DIRECTION ( 'NONE',  ( -1.000000000000000000, 4.190823558986610327E-31, -1.733449886265890494E-32 ) ) ;
#4835=EDGE_LOOP ( 'NONE', ( #21035, #15370, #2143, #8716 ) ) ;
#4860=ORIENTED_EDGE ( 'NONE', *, *, #11239, .T. ) ;
#4872=DIRECTION ( 'NONE',  ( 0.000000000000000000, 0.000000000000000000, 1.000000000000000000 ) ) ;
#4885=CARTESIAN_POINT ( 'NONE',  ( 42.50000000000014921, 8.000000000000003553, -0.4999999999999726885 ) ) ;
#4892=ORIENTED_EDGE ( 'NONE', *, *, #14586, .F. ) ;
#4906=CARTESIAN_POINT ( 'NONE',  ( 0.000000000000000000, 10.49999999999999822, -10.86602540378443749 ) ) ;
#4925=DIRECTION ( 'NONE',  ( -4.190823558986625216E-31, 1.000000000000000000, -4.190823558986625216E-31 ) ) ;
#4930=DIRECTION ( 'NONE',  ( 1.000000000000000000, 0.000000000000000000, 0.000000000000000000 ) ) ;
#4943=CARTESIAN_POINT ( 'NONE',  ( 0.000000000000000000, 0.000000000000000000, 0.000000000000000000 ) ) ;
#4968=DIRECTION ( 'NONE',  ( 0.000000000000000000, -1.387778780781440785E-14, 1.000000000000000000 ) ) ;
#4972=CARTESIAN_POINT ( 'NONE',  ( 37.00000000000014211, 0.000000000000000000, -3.000000000000002665 ) ) ;
#4977=ORIENTED_EDGE ( 'NONE', *, *, #12114, .T. ) ;
#4985=ORIENTED_EDGE ( 'NONE', *, *, #3933, .F. ) ;
#5000=CARTESIAN_POINT ( 'NONE',  ( 37.86602540378461157, 11.00000000000000000, -10.86602540378450676 ) ) ;
#5012=ORIENTED_EDGE ( 'NONE', *, *, #9614, .F. ) ;
#5036=CARTESIAN_POINT ( 'NONE',  ( 42.00000000000014921, 0.5000000000000143219, 2.500000000000030198 ) ) ;
#5046=VERTEX_POINT ( 'NONE', #6552 ) ;
#5063=FACE_OUTER_BOUND ( 'NONE', #7224, .T. ) ;
#5070=ADVANCED_FACE ( 'NONE', ( #4659 ), #3254, .T. ) ;
#5086=CARTESIAN_POINT ( 'NONE',  ( 2.775557561562891351E-14, 0.000000000000000000, -6.499999999999950262 ) ) ;
#5094=DIRECTION ( 'NONE',  ( -0.8660254037844401509, -0.4999999999999977240, 0.000000000000000000 ) ) ;
#5099=CIRCLE ( 'NONE', #10360, 3.000000000000011102 ) ;
#5113=DIRECTION ( 'NONE',  ( 0.000000000000000000, 0.000000000000000000, 1.000000000000000000 ) ) ;
#5132=ORIENTED_EDGE ( 'NONE', *, *, #12227, .F. ) ;
#5142=DIRECTION ( 'NONE',  ( -4.190823558986625216E-31, 1.000000000000000000, -4.190823558986625216E-31 ) ) ;
#5169=CIRCLE ( 'NONE', #17179, 0.5000000000000022204 ) ;
#5209=DIRECTION ( 'NONE',  ( 1.000000000000000000, -4.190823558986621713E-31, 0.000000000000000000 ) ) ;
#5242=EDGE_CURVE ( 'NONE', #13739, #7712, #18979, .T. ) ;
#5258=CARTESIAN_POINT ( 'NONE',  ( 37.43301270189239460, 0.2500000000000002220, -2.999999999999988898 ) ) ;
#5266=LINE ( 'NONE', #23155, #20066 ) ;
#5269=DIRECTION ( 'NONE',  ( -1.000000000000000000, 4.190823558986610327E-31, -1.733449886265890494E-32 ) ) ;
#5289=CARTESIAN_POINT ( 'NONE',  ( 42.50000000000020606, 8.000000000000003553, 5.551115123125782702E-14 ) ) ;
#5295=DIRECTION ( 'NONE',  ( 1.000000000000000000, -4.190823558986610327E-31, 1.733449886265890494E-32 ) ) ;
#5301=DIRECTION ( 'NONE',  ( 0.000000000000000000, 0.000000000000000000, 1.000000000000000000 ) ) ;
#5303=CARTESIAN_POINT ( 'NONE',  ( 37.00000000000017053, 0.2500000000000002220, -2.566987298107781257 ) ) ;
#5306=DIRECTION ( 'NONE',  ( 1.000000000000000000, 0.000000000000000000, 0.000000000000000000 ) ) ;
#5339=VERTEX_POINT ( 'NONE', #4624 ) ;
#5377=CIRCLE ( 'NONE', #21142, 6.000000000000023093 ) ;
#5378=AXIS2_PLACEMENT_3D ( 'NONE', #14750, #14870, #12635 ) ;
#5379=CIRCLE ( 'NONE', #20008, 0.5000000000000017764 ) ;
#5382=EDGE_CURVE ( 'NONE', #12862, #4498, #14352, .T. ) ;
#5385=DIRECTION ( 'NONE',  ( 1.000000000000000000, 0.000000000000000000, 0.000000000000000000 ) ) ;
#5399=CARTESIAN_POINT ( 'NONE',  ( 37.54332536350037230, 10.88440674090231752, -10.22062532321614192 ) ) ;
#5401=FACE_OUTER_BOUND ( 'NONE', #423, .T. ) ;
#5402=DIRECTION ( 'NONE',  ( -1.000000000000000000, 4.437342591868175641E-31, -3.330669073875457788E-16 ) ) ;
#5445=ADVANCED_FACE ( 'NONE', ( #16363 ), #16132, .F. ) ;
#5467=ORIENTED_EDGE ( 'NONE', *, *, #21293, .F. ) ;
#5512=AXIS2_PLACEMENT_3D ( 'NONE', #16534, #14669, #21852 ) ;
#5513=EDGE_CURVE ( 'NONE', #14796, #7570, #17805, .T. ) ;
#5526=ADVANCED_FACE ( 'NONE', ( #17671 ), #1562, .F. ) ;
#5534=CARTESIAN_POINT ( 'NONE',  ( 42.50000000000014921, 2.499999999999995115, -0.4999999999999726885 ) ) ;
#5573=CIRCLE ( 'NONE', #18705, 9.000000000000031974 ) ;
#5580=VECTOR ( 'NONE', #18612, 1000.000000000000000 ) ;
#5605=CARTESIAN_POINT ( 'NONE',  ( 37.86602540378474657, 11.00000000000000533, -2.133974596215531427 ) ) ;
#5610=ORIENTED_EDGE ( 'NONE', *, *, #19725, .F. ) ;
#5615=ORIENTED_EDGE ( 'NONE', *, *, #8507, .T. ) ;
#5626=LINE ( 'NONE', #15840, #3311 ) ;
#5627=AXIS2_PLACEMENT_3D ( 'NONE', #2885, #13043, #20667 ) ;
#5630=CARTESIAN_POINT ( 'NONE',  ( 37.42127086598692642, 0.2176602893534504424, -10.42127086598688912 ) ) ;
#5636=ADVANCED_FACE ( 'NONE', ( #20368 ), #863, .T. ) ;
#5648=DIRECTION ( 'NONE',  ( 0.000000000000000000, 0.000000000000000000, -1.000000000000000000 ) ) ;
#5658=CARTESIAN_POINT ( 'NONE',  ( 37.00000000000017053, 0.2500000000000002220, -2.566987298107781257 ) ) ;
#5670=ADVANCED_FACE ( 'NONE', ( #15530 ), #3072, .F. ) ;
#5672=CARTESIAN_POINT ( 'NONE',  ( 37.86602540378466841, -1.973247953923618070E-14, -2.133974596215482578 ) ) ;
#5687=DIRECTION ( 'NONE',  ( -1.733449886265891589E-32, 4.190823558986610327E-31, -1.000000000000000000 ) ) ;
#5705=DIRECTION ( 'NONE',  ( 0.000000000000000000, -0.5000000000000017764, 0.8660254037844375974 ) ) ;
#5713=CIRCLE ( 'NONE', #21503, 0.5000000000000004441 ) ;
#5718=CARTESIAN_POINT ( 'NONE',  ( 37.60054931026106573, 10.94797865062592024, -2.399450689738686027 ) ) ;
#5733=VECTOR ( 'NONE', #23109, 1000.000000000000000 ) ;
#5776=TOROIDAL_SURFACE ( 'NONE', #20417, 4.366025403784441039, 0.5000000000000000000 ) ;
#5788=CARTESIAN_POINT ( 'NONE',  ( 37.22062532321634620, 0.1155932590976544300, -2.456674636499718289 ) ) ;
#5790=( BOUNDED_CURVE ( )  B_SPLINE_CURVE ( 3, ( #17887, #1536, #19408, #18008 ),
 .UNSPECIFIED., .F., .T. ) 
 B_SPLINE_CURVE_WITH_KNOTS ( ( 4, 4 ),
 ( 3.665191429188060734, 4.712388980384689674 ),
 .UNSPECIFIED. ) 
 CURVE ( )  GEOMETRIC_REPRESENTATION_ITEM ( )  RATIONAL_B_SPLINE_CURVE ( ( 1.000000000000000000, 0.9106836025229538834, 0.9106836025229538834, 1.000000000000000000 ) ) 
 REPRESENTATION_ITEM ( '' )  );
#5792=VECTOR ( 'NONE', #10731, 1000.000000000000000 ) ;
#5799=EDGE_CURVE ( 'NONE', #6309, #17226, #12464, .T. ) ;
#5802=DIRECTION ( 'NONE',  ( 1.733449886265891589E-32, -4.190823558986610327E-31, 1.000000000000000000 ) ) ;
#5820=ADVANCED_FACE ( 'NONE', ( #3543 ), #14955, .F. ) ;
#5823=ORIENTED_EDGE ( 'NONE', *, *, #22327, .F. ) ;
#5835=FACE_OUTER_BOUND ( 'NONE', #599, .T. ) ;
#5842=CARTESIAN_POINT ( 'NONE',  ( 37.48161866288229760, 10.82270004028423571, -2.902788078020195339 ) ) ;
#5849=ORIENTED_EDGE ( 'NONE', *, *, #17867, .T. ) ;
#5853=LINE ( 'NONE', #13017, #11358 ) ;
#5888=ORIENTED_EDGE ( 'NONE', *, *, #1966, .F. ) ;
#5903=CARTESIAN_POINT ( 'NONE',  ( 37.00000000000011369, 11.00000000000000000, -10.00000000000000888 ) ) ;
#5906=VECTOR ( 'NONE', #6749, 1000.000000000000000 ) ;
#5918=EDGE_CURVE ( 'NONE', #15879, #16689, #12504, .T. ) ;
#5924=DIRECTION ( 'NONE',  ( 4.190823558986625216E-31, -1.000000000000000000, 4.190823558986625216E-31 ) ) ;
#5926=ORIENTED_EDGE ( 'NONE', *, *, #12130, .T. ) ;
#5936=EDGE_CURVE ( 'NONE', #15879, #13703, #7415, .T. ) ;
#5953=EDGE_CURVE ( 'NONE', #7570, #22556, #3696, .T. ) ;
#5960=ORIENTED_EDGE ( 'NONE', *, *, #23080, .F. ) ;
#5991=EDGE_CURVE ( 'NONE', #16286, #13739, #18583, .T. ) ;
#6004=CARTESIAN_POINT ( 'NONE',  ( 2.775557561562891351E-14, 0.000000000000000000, -6.499999999999950262 ) ) ;
#6029=CARTESIAN_POINT ( 'NONE',  ( 42.50000000000014921, 8.500000000000003553, -0.4999999999999726885 ) ) ;
#6034=ORIENTED_EDGE ( 'NONE', *, *, #16204, .F. ) ;
#6036=UNCERTAINTY_MEASURE_WITH_UNIT (LENGTH_MEASURE( 1.000000000000000082E-05 ), #11281, 'distance_accuracy_value', 'NONE');
#6041=ORIENTED_EDGE ( 'NONE', *, *, #5936, .F. ) ;
#6042=LINE ( 'NONE', #11437, #7260 ) ;
#6062=ORIENTED_EDGE ( 'NONE', *, *, #12821, .T. ) ;
#6074=DIRECTION ( 'NONE',  ( -1.000000000000000000, -1.374679200952735400E-16, -3.676447422453419544E-32 ) ) ;
#6086=DIRECTION ( 'NONE',  ( -1.000000000000000000, 4.190823558986610327E-31, -1.733449886265890494E-32 ) ) ;
#6105=CARTESIAN_POINT ( 'NONE',  ( 2.775557561562891351E-14, 10.49999999999999822, -6.499999999999950262 ) ) ;
#6127=CARTESIAN_POINT ( 'NONE',  ( 5.551115123125782702E-14, 3.000000000000027089, 2.500000000000071498 ) ) ;
#6139=CARTESIAN_POINT ( 'NONE',  ( 42.50000000000014921, 8.000000000000003553, -0.4999999999999726885 ) ) ;
#6150=ORIENTED_EDGE ( 'NONE', *, *, #6796, .T. ) ;
#6179=CARTESIAN_POINT ( 'NONE',  ( 42.00000000000014921, 11.00000000000000000, -0.4999999999999449329 ) ) ;
#6196=EDGE_CURVE ( 'NONE', #18871, #13205, #15159, .T. ) ;
#6205=CARTESIAN_POINT ( 'NONE',  ( 37.69139372032820745, 3.387530319305491578E-14, -10.77870956205554975 ) ) ;
#6227=FACE_OUTER_BOUND ( 'NONE', #14200, .T. ) ;
#6252=CARTESIAN_POINT ( 'NONE',  ( 37.68301270189238750, -2.676886543277417521E-15, -10.50000000000003908 ) ) ;
#6264=ORIENTED_EDGE ( 'NONE', *, *, #3933, .T. ) ;
#6298=AXIS2_PLACEMENT_3D ( 'NONE', #20581, #4326, #15036 ) ;
#6309=VERTEX_POINT ( 'NONE', #14450 ) ;
#6323=PRESENTATION_STYLE_ASSIGNMENT (( #20803 ) ) ;
#6328=ADVANCED_FACE ( 'NONE', ( #5401 ), #15963, .T. ) ;
#6334=CARTESIAN_POINT ( 'NONE',  ( 37.00000000000014211, 0.000000000000000000, -3.000000000000002665 ) ) ;
#6335=ORIENTED_EDGE ( 'NONE', *, *, #4067, .F. ) ;
#6369=CARTESIAN_POINT ( 'NONE',  ( 42.00000000000014921, 8.000000000000003553, -15.00000000000001421 ) ) ;
#6390=VERTEX_POINT ( 'NONE', #6179 ) ;
#6443=VERTEX_POINT ( 'NONE', #999 ) ;
#6465=ORIENTED_EDGE ( 'NONE', *, *, #5513, .F. ) ;
#6498=EDGE_LOOP ( 'NONE', ( #19056, #15341, #22145, #7003 ) ) ;
#6506=CIRCLE ( 'NONE', #14455, 0.5000000000000017764 ) ;
#6552=CARTESIAN_POINT ( 'NONE',  ( 42.50000000000020606, 2.999999999999999112, 5.551115123125782702E-14 ) ) ;
#6565=CLOSED_SHELL ( 'NONE', ( #15538, #16429, #21425, #18151, #12028, #9072, #8965, #19303, #7525, #10249, #12846, #1605, #222, #22483, #11251, #5636, #14567, #12067, #14106, #18438, #5445, #18139, #3413, #12359, #11997, #337, #13861, #21460, #19463, #14837, #1069, #5526, #473, #19281, #5670, #1591, #10545, #10280, #3518, #20895, #5820, #11442, #18588, #11133, #23110, #10309, #21766, #4331, #3623, #8681, #6328, #16172, #15187, #9255, #20326, #5070, #3182 ) ) ;
#6582=DIRECTION ( 'NONE',  ( -4.190823558986625216E-31, 1.000000000000000000, -4.190823558986625216E-31 ) ) ;
#6608=ORIENTED_EDGE ( 'NONE', *, *, #6796, .F. ) ;
#6622=CARTESIAN_POINT ( 'NONE',  ( 37.00000000000014211, 0.000000000000000000, -3.000000000000002665 ) ) ;
#6626=ORIENTED_EDGE ( 'NONE', *, *, #6196, .F. ) ;
#6635=EDGE_CURVE ( 'NONE', #7856, #13205, #17807, .T. ) ;
#6637=VECTOR ( 'NONE', #20818, 1000.000000000000000 ) ;
#6683=CARTESIAN_POINT ( 'NONE',  ( 42.00000000000014921, 11.00000000000000000, -12.50000000000005329 ) ) ;
#6702=ORIENTED_EDGE ( 'NONE', *, *, #12164, .F. ) ;
#6707=ORIENTED_EDGE ( 'NONE', *, *, #23182, .F. ) ;
#6730=ORIENTED_EDGE ( 'NONE', *, *, #3786, .F. ) ;
#6739=DIRECTION ( 'NONE',  ( -4.190823558986625216E-31, 1.000000000000000000, -4.190823558986625216E-31 ) ) ;
#6749=DIRECTION ( 'NONE',  ( 1.733449886265891589E-32, -4.190823558986610327E-31, 1.000000000000000000 ) ) ;
#6771=EDGE_CURVE ( 'NONE', #16034, #15424, #20580, .T. ) ;
#6796=EDGE_CURVE ( 'NONE', #2883, #14796, #22020, .T. ) ;
#6799=CARTESIAN_POINT ( 'NONE',  ( 2.775557561562891351E-14, 8.000000000000003553, -12.50000000000001066 ) ) ;
#6802=DIRECTION ( 'NONE',  ( 1.000000000000000000, -4.437342591868175641E-31, 3.330669073875457788E-16 ) ) ;
#6820=ORIENTED_EDGE ( 'NONE', *, *, #18576, .T. ) ;
#6841=AXIS2_PLACEMENT_3D ( 'NONE', #15952, #12899, #16409 ) ;
#6843=ORIENTED_EDGE ( 'NONE', *, *, #18170, .T. ) ;
#6877=ORIENTED_EDGE ( 'NONE', *, *, #591, .F. ) ;
#6880=CIRCLE ( 'NONE', #13646, 0.5000000000000017764 ) ;
#6885=CARTESIAN_POINT ( 'NONE',  ( 42.50000000000014921, 2.999999999999999112, -0.4999999999999726885 ) ) ;
#6889=CYLINDRICAL_SURFACE ( 'NONE', #9493, 0.5000000000000017764 ) ;
#6933=CIRCLE ( 'NONE', #9561, 6.000000000000022204 ) ;
#6940=EDGE_CURVE ( 'NONE', #7345, #3408, #20729, .T. ) ;
#6955=FACE_OUTER_BOUND ( 'NONE', #15070, .T. ) ;
#6974=AXIS2_PLACEMENT_3D ( 'NONE', #4708, #17045, #10005 ) ;
#6977=EDGE_LOOP ( 'NONE', ( #15941, #2722, #22874, #6843 ) ) ;
#6993=DIRECTION ( 'NONE',  ( 1.000000000000000000, -4.190823558986610327E-31, 1.733449886265890494E-32 ) ) ;
#6995=DIRECTION ( 'NONE',  ( 0.000000000000000000, 0.000000000000000000, 1.000000000000000000 ) ) ;
#7003=ORIENTED_EDGE ( 'NONE', *, *, #4398, .F. ) ;
#7015=AXIS2_PLACEMENT_3D ( 'NONE', #17866, #5402, #12321 ) ;
#7016=DIRECTION ( 'NONE',  ( -1.000000000000000000, 4.190823558986610327E-31, -1.733449886265890494E-32 ) ) ;
#7022=FACE_OUTER_BOUND ( 'NONE', #9919, .T. ) ;
#7027=CARTESIAN_POINT ( 'NONE',  ( 2.775557561562891351E-14, 0.5000000000000004441, -3.000000000000002665 ) ) ;
#7036=LINE ( 'NONE', #1836, #9921 ) ;
#7043=CARTESIAN_POINT ( 'NONE',  ( 2.775557561562891351E-14, 10.99999999999998579, -0.4999999999999865663 ) ) ;
#7047=CARTESIAN_POINT ( 'NONE',  ( 37.57823792062862367, 10.91119608832010890, -10.29045043747236754 ) ) ;
#7081=CARTESIAN_POINT ( 'NONE',  ( 37.52451905283851374, 10.90849364905388974, -2.816987298107761273 ) ) ;
#7098=EDGE_LOOP ( 'NONE', ( #19108, #19342, #4135, #16977 ) ) ;
#7154=EDGE_LOOP ( 'NONE', ( #8420, #21242, #977, #60 ) ) ;
#7197=VERTEX_POINT ( 'NONE', #471 ) ;
#7214=CARTESIAN_POINT ( 'NONE',  ( 42.50000000000017764, 0.5000000000000143219, 2.500000000000071498 ) ) ;
#7224=EDGE_LOOP ( 'NONE', ( #9916, #4145, #20857, #11267 ) ) ;
#7249=CARTESIAN_POINT ( 'NONE',  ( 37.43301270189233776, 10.75000000000000000, -9.999999999999994671 ) ) ;
#7252=ORIENTED_EDGE ( 'NONE', *, *, #9695, .T. ) ;
#7258=VECTOR ( 'NONE', #18894, 1000.000000000000000 ) ;
#7260=VECTOR ( 'NONE', #20046, 1000.000000000000000 ) ;
#7272=AXIS2_PLACEMENT_3D ( 'NONE', #21336, #12370, #19553 ) ;
#7281=CARTESIAN_POINT ( 'NONE',  ( 37.04362427881607545, 10.78777973366380216, -10.45482484129298051 ) ) ;
#7303=DIRECTION ( 'NONE',  ( 0.000000000000000000, 0.000000000000000000, 1.000000000000000000 ) ) ;
#7340=EDGE_CURVE ( 'NONE', #180, #5339, #19483, .T. ) ;
#7345=VERTEX_POINT ( 'NONE', #15506 ) ;
#7363=CARTESIAN_POINT ( 'NONE',  ( 37.09721192198001916, 10.82270004028423394, -2.518381337117829410 ) ) ;
#7378=DIRECTION ( 'NONE',  ( 0.000000000000000000, 0.000000000000000000, 1.000000000000000000 ) ) ;
#7388=CARTESIAN_POINT ( 'NONE',  ( 37.09721192198001916, 0.1772999597158308738, -10.48161866288212885 ) ) ;
#7402=LINE ( 'NONE', #7742, #12248 ) ;
#7415=LINE ( 'NONE', #19994, #19464 ) ;
#7431=CARTESIAN_POINT ( 'NONE',  ( 37.57823792062836787, 0.08880391168000995039, -2.709549562527593825 ) ) ;
#7464=DIRECTION ( 'NONE',  ( -0.4472135954999518215, 0.7745966692414842925, 0.4472135954999624796 ) ) ;
#7482=ORIENTED_EDGE ( 'NONE', *, *, #8881, .F. ) ;
#7524=CARTESIAN_POINT ( 'NONE',  ( -2.775557561562891351E-14, 10.74999999999998579, -2.566987298107781257 ) ) ;
#7525=ADVANCED_FACE ( 'NONE', ( #13151 ), #9388, .T. ) ;
#7540=ORIENTED_EDGE ( 'NONE', *, *, #19570, .T. ) ;
#7570=VERTEX_POINT ( 'NONE', #14792 ) ;
#7573=ORIENTED_EDGE ( 'NONE', *, *, #11395, .F. ) ;
#7579=CARTESIAN_POINT ( 'NONE',  ( 37.86602540378459025, -1.387778780781445676E-14, -2.133974596215476360 ) ) ;
#7595=EDGE_LOOP ( 'NONE', ( #6465, #19424, #7482, #15236 ) ) ;
#7600=ORIENTED_EDGE ( 'NONE', *, *, #19893, .T. ) ;
#7603=CARTESIAN_POINT ( 'NONE',  ( 0.000000000000000000, 10.49999999999999822, -10.86602540378443749 ) ) ;
#7642=DIRECTION ( 'NONE',  ( 0.000000000000000000, -4.190823558986609452E-31, 1.000000000000000000 ) ) ;
#7682=AXIS2_PLACEMENT_3D ( 'NONE', #3426, #9058, #17890 ) ;
#7690=EDGE_CURVE ( 'NONE', #6390, #16034, #13497, .T. ) ;
#7703=CARTESIAN_POINT ( 'NONE',  ( 2.775557561562891351E-14, 8.000000000000003553, -6.499999999999950262 ) ) ;
#7705=CARTESIAN_POINT ( 'NONE',  ( 37.36637401601559105, 10.68627026436968386, -2.633625983984380081 ) ) ;
#7709=VERTEX_POINT ( 'NONE', #7027 ) ;
#7712=VERTEX_POINT ( 'NONE', #5258 ) ;
#7717=DIRECTION ( 'NONE',  ( 0.000000000000000000, 0.000000000000000000, 1.000000000000000000 ) ) ;
#7734=ORIENTED_EDGE ( 'NONE', *, *, #11395, .T. ) ;
#7742=CARTESIAN_POINT ( 'NONE',  ( 0.000000000000000000, 1.387778780781445676E-14, -10.86602540378443749 ) ) ;
#7765=CARTESIAN_POINT ( 'NONE',  ( 37.77870956205638464, -7.009096939670001340E-15, -2.308606279672925865 ) ) ;
#7766=EDGE_CURVE ( 'NONE', #22878, #12541, #19833, .T. ) ;
#7780=VECTOR ( 'NONE', #11306, 1000.000000000000000 ) ;
#7802=AXIS2_PLACEMENT_3D ( 'NONE', #14557, #17625, #17742 ) ;
#7828=ORIENTED_EDGE ( 'NONE', *, *, #17867, .F. ) ;
#7830=ORIENTED_EDGE ( 'NONE', *, *, #10067, .T. ) ;
#7845=CIRCLE ( 'NONE', #8995, 0.5000000000000017764 ) ;
#7848=CARTESIAN_POINT ( 'NONE',  ( 37.34641016151398674, 0.3999999999999195310, -10.34641016151375581 ) ) ;
#7856=VERTEX_POINT ( 'NONE', #14529 ) ;
#7873=CARTESIAN_POINT ( 'NONE',  ( 2.775557561562891351E-14, 7.999999999999983125, -0.4999999999999865663 ) ) ;
#7897=DIRECTION ( 'NONE',  ( -1.000000000000000000, 4.190823558986610327E-31, -1.733449886265890494E-32 ) ) ;
#7911=ORIENTED_EDGE ( 'NONE', *, *, #14558, .F. ) ;
#7921=CARTESIAN_POINT ( 'NONE',  ( 37.86602540378461157, 10.49999999999999822, -6.500000000000005329 ) ) ;
#7950=ORIENTED_EDGE ( 'NONE', *, *, #22210, .F. ) ;
#7952=CARTESIAN_POINT ( 'NONE',  ( 37.43301270189239460, 0.2500000000000002220, -6.500000000000019540 ) ) ;
#7956=DIRECTION ( 'NONE',  ( 4.190823558986625216E-31, -1.000000000000000000, 4.190823558986625216E-31 ) ) ;
#7973=CARTESIAN_POINT ( 'NONE',  ( 0.000000000000000000, 0.5000000000000108802, -10.86602540378443749 ) ) ;
#8004=FACE_OUTER_BOUND ( 'NONE', #11605, .T. ) ;
#8020=AXIS2_PLACEMENT_3D ( 'NONE', #2586, #4925, #13414 ) ;
#8021=DIRECTION ( 'NONE',  ( 1.733449886265891589E-32, -4.190823558986610327E-31, 1.000000000000000000 ) ) ;
#8089=FACE_OUTER_BOUND ( 'NONE', #11365, .T. ) ;
#8101=DIRECTION ( 'NONE',  ( 1.733449886265891589E-32, -4.190823558986610327E-31, 1.000000000000000000 ) ) ;
#8154=DIRECTION ( 'NONE',  ( 4.190823558986621713E-31, 1.000000000000000000, 4.190823558986611203E-31 ) ) ;
#8191=AXIS2_PLACEMENT_3D ( 'NONE', #4906, #3167, #1394 ) ;
#8208=EDGE_LOOP ( 'NONE', ( #862, #633, #4193 ) ) ;
#8260=EDGE_CURVE ( 'NONE', #12892, #7709, #5379, .T. ) ;
#8276=AXIS2_PLACEMENT_3D ( 'NONE', #1582, #14057, #4872 ) ;
#8321=EDGE_LOOP ( 'NONE', ( #15628, #3028, #12153 ) ) ;
#8323=DIRECTION ( 'NONE',  ( 1.000000000000000000, -4.190823558986621713E-31, 0.000000000000000000 ) ) ;
#8360=AXIS2_PLACEMENT_3D ( 'NONE', #13316, #20499, #4351 ) ;
#8364=( BOUNDED_CURVE ( )  B_SPLINE_CURVE ( 3, ( #1193, #17400, #6252, #11526 ),
 .UNSPECIFIED., .F., .T. ) 
 B_SPLINE_CURVE_WITH_KNOTS ( ( 4, 4 ),
 ( 3.665191429188050076, 4.712388980384689674 ),
 .UNSPECIFIED. ) 
 CURVE ( )  GEOMETRIC_REPRESENTATION_ITEM ( )  RATIONAL_B_SPLINE_CURVE ( ( 1.000000000000000000, 0.9106836025229521070, 0.9106836025229521070, 1.000000000000000000 ) ) 
 REPRESENTATION_ITEM ( '' )  );
#8380=EDGE_LOOP ( 'NONE', ( #21504, #481, #16404, #2117 ) ) ;
#8382=ORIENTED_EDGE ( 'NONE', *, *, #4338, .F. ) ;
#8383=DIRECTION ( 'NONE',  ( -1.000000000000000000, 4.190823558986610327E-31, -1.733449886265890494E-32 ) ) ;
#8420=ORIENTED_EDGE ( 'NONE', *, *, #10863, .T. ) ;
#8421=ORIENTED_EDGE ( 'NONE', *, *, #13569, .F. ) ;
#8450=EDGE_LOOP ( 'NONE', ( #18392, #13560, #5888, #15770 ) ) ;
#8456=CARTESIAN_POINT ( 'NONE',  ( 42.00000000000017764, 5.500000000000001776, 2.000000000000057288 ) ) ;
#8473=DIRECTION ( 'NONE',  ( 0.000000000000000000, 0.000000000000000000, -1.000000000000000000 ) ) ;
#8502=CARTESIAN_POINT ( 'NONE',  ( 2.775557561562891351E-14, 2.999999999999999112, -12.50000000000001066 ) ) ;
#8507=EDGE_CURVE ( 'NONE', #9447, #15190, #6042, .T. ) ;
#8521=EDGE_CURVE ( 'NONE', #1669, #19695, #3489, .T. ) ;
#8524=ORIENTED_EDGE ( 'NONE', *, *, #10798, .F. ) ;
#8579=AXIS2_PLACEMENT_3D ( 'NONE', #4303, #18552, #20323 ) ;
#8589=DIRECTION ( 'NONE',  ( 1.733449886265891589E-32, -4.190823558986610327E-31, 1.000000000000000000 ) ) ;
#8625=DIRECTION ( 'NONE',  ( 1.000000000000000000, -4.190823558986621713E-31, 0.000000000000000000 ) ) ;
#8681=ADVANCED_FACE ( 'NONE', ( #15548 ), #14013, .T. ) ;
#8686=CARTESIAN_POINT ( 'NONE',  ( 42.00000000000020606, 2.999999999999999112, -15.50000000000004086 ) ) ;
#8690=DIRECTION ( 'NONE',  ( 1.000000000000000000, -4.437342591868175641E-31, 3.330669073875457788E-16 ) ) ;
#8708=CYLINDRICAL_SURFACE ( 'NONE', #18816, 0.5000000000000004441 ) ;
#8716=ORIENTED_EDGE ( 'NONE', *, *, #14877, .F. ) ;
#8726=EDGE_LOOP ( 'NONE', ( #9679, #17563, #19228, #19810 ) ) ;
#8739=DIRECTION ( 'NONE',  ( 0.000000000000000000, 0.000000000000000000, -1.000000000000000000 ) ) ;
#8743=DIRECTION ( 'NONE',  ( -4.190823558986625216E-31, 1.000000000000000000, -4.190823558986625216E-31 ) ) ;
#8749=EDGE_LOOP ( 'NONE', ( #15920, #3084, #3461, #12124 ) ) ;
#8800=DIRECTION ( 'NONE',  ( 1.000000000000000000, -4.190823558986610327E-31, 1.733449886265890494E-32 ) ) ;
#8804=CARTESIAN_POINT ( 'NONE',  ( 37.09721192198001916, 10.82270004028415933, -10.48161866288213240 ) ) ;
#8813=CARTESIAN_POINT ( 'NONE',  ( 2.775557561562891351E-14, 10.49999999999999822, -9.999999999999968026 ) ) ;
#8832=DIRECTION ( 'NONE',  ( -1.000000000000000000, 4.190823558986610327E-31, -1.733449886265890494E-32 ) ) ;
#8835=FACE_OUTER_BOUND ( 'NONE', #21729, .T. ) ;
#8861=DIRECTION ( 'NONE',  ( 3.330669073875457788E-16, 0.000000000000000000, -1.000000000000000000 ) ) ;
#8881=EDGE_CURVE ( 'NONE', #15190, #17995, #2469, .T. ) ;
#8899=ORIENTED_EDGE ( 'NONE', *, *, #1966, .T. ) ;
#8906=VERTEX_POINT ( 'NONE', #14704 ) ;
#8911=CARTESIAN_POINT ( 'NONE',  ( 42.00000000000020606, 8.000000000000003553, -0.4999999999999449329 ) ) ;
#8939=CARTESIAN_POINT ( 'NONE',  ( 42.50000000000014921, 8.000000000000003553, -12.49999999999998401 ) ) ;
#8963=ORIENTED_EDGE ( 'NONE', *, *, #393, .F. ) ;
#8965=ADVANCED_FACE ( 'NONE', ( #11181 ), #485, .F. ) ;
#8995=AXIS2_PLACEMENT_3D ( 'NONE', #14185, #3377, #19590 ) ;
#8998=EDGE_LOOP ( 'NONE', ( #16030, #5132, #11955, #6702 ) ) ;
#9033=CARTESIAN_POINT ( 'NONE',  ( 42.50000000000020606, 2.499999999999998668, -13.00000000000002487 ) ) ;
#9054=CARTESIAN_POINT ( 'NONE',  ( 42.50000000000014921, 2.999999999999999112, -12.49999999999998401 ) ) ;
#9058=DIRECTION ( 'NONE',  ( -4.190823558986625216E-31, 1.000000000000000000, -4.190823558986625216E-31 ) ) ;
#9062=ORIENTED_EDGE ( 'NONE', *, *, #17515, .F. ) ;
#9071=CARTESIAN_POINT ( 'NONE',  ( 37.00000000000027711, 0.2500000000000007216, -2.566987298107707982 ) ) ;
#9072=ADVANCED_FACE ( 'NONE', ( #8004 ), #10221, .F. ) ;
#9075=FACE_OUTER_BOUND ( 'NONE', #19286, .T. ) ;
#9082=FACE_OUTER_BOUND ( 'NONE', #7595, .T. ) ;
#9084=DIRECTION ( 'NONE',  ( 0.000000000000000000, 0.000000000000000000, -1.000000000000000000 ) ) ;
#9088=AXIS2_PLACEMENT_3D ( 'NONE', #16526, #435, #21967 ) ;
#9143=CIRCLE ( 'NONE', #7272, 3.000000000000011102 ) ;
#9156=CARTESIAN_POINT ( 'NONE',  ( 37.04362427881591202, 0.2122202663360315822, -10.45482484129306400 ) ) ;
#9175=DIRECTION ( 'NONE',  ( -1.000000000000000000, 4.190823558986610327E-31, -1.733449886265890494E-32 ) ) ;
#9180=DIRECTION ( 'NONE',  ( 0.000000000000000000, 0.000000000000000000, -1.000000000000000000 ) ) ;
#9195=CARTESIAN_POINT ( 'NONE',  ( 37.54332536350039362, 0.1155932590976206792, -2.779374676783886056 ) ) ;
#9224=VERTEX_POINT ( 'NONE', #5289 ) ;
#9227=AXIS2_PLACEMENT_3D ( 'NONE', #1076, #18706, #18946 ) ;
#9238=CARTESIAN_POINT ( 'NONE',  ( 37.42127086598728170, 10.78233971064650731, -2.578729134013173940 ) ) ;
#9255=ADVANCED_FACE ( 'NONE', ( #1526 ), #18925, .T. ) ;
#9257=DIRECTION ( 'NONE',  ( -1.000000000000000000, -8.030776666391858360E-17, -3.330669073875458281E-16 ) ) ;
#9273=ORIENTED_EDGE ( 'NONE', *, *, #14656, .T. ) ;
#9295=( NAMED_UNIT ( * ) PLANE_ANGLE_UNIT ( ) SI_UNIT ( $, .RADIAN. ) );
#9304=EDGE_LOOP ( 'NONE', ( #23016, #23094, #9273, #20275 ) ) ;
#9308=CARTESIAN_POINT ( 'NONE',  ( 37.34641016151396542, 0.3999999999999052647, -2.653589838486210883 ) ) ;
#9318=DIRECTION ( 'NONE',  ( 1.000000000000000000, 0.000000000000000000, 0.000000000000000000 ) ) ;
#9319=DIRECTION ( 'NONE',  ( 1.000000000000000000, -4.190823558986610327E-31, 1.733449886265890494E-32 ) ) ;
#9328=LINE ( 'NONE', #4018, #9683 ) ;
#9334=VERTEX_POINT ( 'NONE', #20101 ) ;
#9355=DIRECTION ( 'NONE',  ( 1.000000000000000000, -8.030776666391948340E-17, 3.330669073875457788E-16 ) ) ;
#9357=CARTESIAN_POINT ( 'NONE',  ( 37.86602540378461157, 11.00000000000000533, -2.133974596215514552 ) ) ;
#9372=CARTESIAN_POINT ( 'NONE',  ( 2.775557561562891351E-14, 11.00000000000000000, -6.499999999999950262 ) ) ;
#9388=PLANE ( 'NONE',  #8579 ) ;
#9390=EDGE_CURVE ( 'NONE', #13703, #18075, #2615, .T. ) ;
#9399=DIRECTION ( 'NONE',  ( -1.000000000000000000, 4.437342591868175641E-31, -3.330669073875457788E-16 ) ) ;
#9401=DIRECTION ( 'NONE',  ( 0.000000000000000000, 0.000000000000000000, 1.000000000000000000 ) ) ;
#9412=CARTESIAN_POINT ( 'NONE',  ( 2.775557561562891351E-14, 0.2500000000000106581, -10.43301270189220276 ) ) ;
#9425=CARTESIAN_POINT ( 'NONE',  ( 37.86602540378471815, -1.973247953923618070E-14, -2.133974596215504338 ) ) ;
#9435=DIRECTION ( 'NONE',  ( 0.000000000000000000, 0.000000000000000000, -1.000000000000000000 ) ) ;
#9447=VERTEX_POINT ( 'NONE', #18920 ) ;
#9465=CARTESIAN_POINT ( 'NONE',  ( 37.86602540378459025, -1.387778780781445676E-14, -2.133974596215476360 ) ) ;
#9478=CYLINDRICAL_SURFACE ( 'NONE', #11809, 3.000000000000011546 ) ;
#9493=AXIS2_PLACEMENT_3D ( 'NONE', #3593, #7016, #10527 ) ;
#9503=AXIS2_PLACEMENT_3D ( 'NONE', #21256, #3013, #1479 ) ;
#9539=DIRECTION ( 'NONE',  ( -1.000000000000000000, 4.190823558986610327E-31, -1.733449886265890494E-32 ) ) ;
#9540=CARTESIAN_POINT ( 'NONE',  ( 37.69139372032760349, 2.146704506890337223E-14, -2.221290437944543061 ) ) ;
#9557=CYLINDRICAL_SURFACE ( 'NONE', #20605, 3.000000000000011546 ) ;
#9561=AXIS2_PLACEMENT_3D ( 'NONE', #14374, #1559, #21571 ) ;
#9564=ORIENTED_EDGE ( 'NONE', *, *, #20056, .T. ) ;
#9574=EDGE_LOOP ( 'NONE', ( #15874, #12979, #7911, #20067 ) ) ;
#9579=DIRECTION ( 'NONE',  ( 1.733449886265891589E-32, -4.190823558986610327E-31, 1.000000000000000000 ) ) ;
#9588=CARTESIAN_POINT ( 'NONE',  ( 37.22062532321636752, 10.88440674090231219, -2.456674636499794673 ) ) ;
#9592=ORIENTED_EDGE ( 'NONE', *, *, #14711, .F. ) ;
#9613=CARTESIAN_POINT ( 'NONE',  ( 37.43301270189240171, 0.2499999999999834577, -10.00000000000006573 ) ) ;
#9614=EDGE_CURVE ( 'NONE', #17626, #6390, #18882, .T. ) ;
#9619=COLOUR_RGB ( '', 0.40784314, 0.44705882, 0.49803922) ;
#9628=CARTESIAN_POINT ( 'NONE',  ( 37.86602540378461157, 11.00000000000000000, -2.133974596215532316 ) ) ;
#9652=ORIENTED_EDGE ( 'NONE', *, *, #567, .T. ) ;
#9679=ORIENTED_EDGE ( 'NONE', *, *, #8260, .F. ) ;
#9683=VECTOR ( 'NONE', #11200, 1000.000000000000000 ) ;
#9695=EDGE_CURVE ( 'NONE', #15040, #3943, #5377, .T. ) ;
#9706=AXIS2_PLACEMENT_3D ( 'NONE', #18723, #11654, #2714 ) ;
#9736=DIRECTION ( 'NONE',  ( 0.000000000000000000, -4.190823558986610327E-31, 1.000000000000000000 ) ) ;
#9760=CARTESIAN_POINT ( 'NONE',  ( 37.43301270189236618, 10.75000000000000000, -2.999999999999988898 ) ) ;
#9761=CARTESIAN_POINT ( 'NONE',  ( 37.18301270189234486, 0.09150635094609947673, -2.475480947161597278 ) ) ;
#9777=AXIS2_PLACEMENT_3D ( 'NONE', #8502, #17665, #1556 ) ;
#9823=EDGE_CURVE ( 'NONE', #3943, #16034, #5853, .T. ) ;
#9844=( NAMED_UNIT ( * ) PLANE_ANGLE_UNIT ( ) SI_UNIT ( $, .RADIAN. ) );
#9847=AXIS2_PLACEMENT_3D ( 'NONE', #5903, #21904, #11192 ) ;
#9849=EDGE_LOOP ( 'NONE', ( #5823, #15310, #19839, #22682 ) ) ;
#9851=ORIENTED_EDGE ( 'NONE', *, *, #21677, .F. ) ;
#9907=CARTESIAN_POINT ( 'NONE',  ( 2.775557561562891351E-14, 8.000000000000003553, -12.50000000000001066 ) ) ;
#9908=CARTESIAN_POINT ( 'NONE',  ( 0.000000000000000000, 7.999999999999983125, 0.000000000000000000 ) ) ;
#9916=ORIENTED_EDGE ( 'NONE', *, *, #23063, .F. ) ;
#9919=EDGE_LOOP ( 'NONE', ( #3027, #4221, #10722, #7950 ) ) ;
#9921=VECTOR ( 'NONE', #17486, 1000.000000000000000 ) ;
#9923=EDGE_LOOP ( 'NONE', ( #11468, #20685, #18975, #10000 ) ) ;
#9928=PLANE ( 'NONE',  #14810 ) ;
#9934=CIRCLE ( 'NONE', #19710, 0.5000000000000017764 ) ;
#10000=ORIENTED_EDGE ( 'NONE', *, *, #6635, .F. ) ;
#10005=DIRECTION ( 'NONE',  ( 0.000000000000000000, 0.000000000000000000, -1.000000000000000000 ) ) ;
#10052=ORIENTED_EDGE ( 'NONE', *, *, #19971, .F. ) ;
#10057=AXIS2_PLACEMENT_3D ( 'NONE', #16620, #9355, #12999 ) ;
#10067=EDGE_CURVE ( 'NONE', #14576, #5046, #6880, .T. ) ;
#10079=EDGE_LOOP ( 'NONE', ( #12337, #12880, #17159, #22714, #4490, #16380, #13736, #12825 ) ) ;
#10081=( NAMED_UNIT ( * ) SI_UNIT ( $, .STERADIAN. ) SOLID_ANGLE_UNIT ( ) );
#10115=AXIS2_PLACEMENT_3D ( 'NONE', #16069, #8800, #9401 ) ;
#10130=DIRECTION ( 'NONE',  ( -1.733449886265891589E-32, 4.190823558986610327E-31, -1.000000000000000000 ) ) ;
#10165=ORIENTED_EDGE ( 'NONE', *, *, #19941, .T. ) ;
#10176=DIRECTION ( 'NONE',  ( -1.756300210255732376E-61, 4.190823558986625216E-31, 1.000000000000000000 ) ) ;
#10184=CARTESIAN_POINT ( 'NONE',  ( 37.77870956205668307, 4.228348986099717415E-15, -10.69139372032708124 ) ) ;
#10187=ORIENTED_EDGE ( 'NONE', *, *, #12164, .T. ) ;
#10204=FACE_OUTER_BOUND ( 'NONE', #8998, .T. ) ;
#10221=CYLINDRICAL_SURFACE ( 'NONE', #8020, 6.500000000000023981 ) ;
#10225=CARTESIAN_POINT ( 'NONE',  ( 42.50000000000014921, 8.000000000000003553, -14.99999999999998579 ) ) ;
#10228=FACE_OUTER_BOUND ( 'NONE', #14622, .T. ) ;
#10249=ADVANCED_FACE ( 'NONE', ( #12990 ), #3589, .T. ) ;
#10268=CARTESIAN_POINT ( 'NONE',  ( 42.00000000000014921, 2.999999999999999112, 2.500000000000030198 ) ) ;
#10278=ORIENTED_EDGE ( 'NONE', *, *, #17147, .F. ) ;
#10280=ADVANCED_FACE ( 'NONE', ( #3189 ), #13339, .T. ) ;
#10292=TOROIDAL_SURFACE ( 'NONE', #21948, 3.500000000000001776, 0.5000000000000000000 ) ;
#10294=AXIS2_PLACEMENT_3D ( 'NONE', #12250, #6993, #8739 ) ;
#10303=DIRECTION ( 'NONE',  ( 1.000000000000000000, -4.190823558986610327E-31, 1.733449886265890494E-32 ) ) ;
#10308=ORIENTED_EDGE ( 'NONE', *, *, #18153, .F. ) ;
#10309=ADVANCED_FACE ( 'NONE', ( #10228 ), #1188, .F. ) ;
#10360=AXIS2_PLACEMENT_3D ( 'NONE', #4612, #17430, #4735 ) ;
#10379=DIRECTION ( 'NONE',  ( 0.000000000000000000, 0.000000000000000000, 1.000000000000000000 ) ) ;
#10384=CARTESIAN_POINT ( 'NONE',  ( 2.775557561562891351E-14, 8.000000000000003553, -6.499999999999950262 ) ) ;
#10421=DIRECTION ( 'NONE',  ( 1.756300210255732376E-61, -4.190823558986625216E-31, -1.000000000000000000 ) ) ;
#10428=ORIENTED_EDGE ( 'NONE', *, *, #11022, .T. ) ;
#10435=EDGE_LOOP ( 'NONE', ( #17538, #10777, #2003, #10052 ) ) ;
#10437=DIRECTION ( 'NONE',  ( 1.733449886265891589E-32, -4.190823558986610327E-31, 1.000000000000000000 ) ) ;
#10475=( GEOMETRIC_REPRESENTATION_CONTEXT ( 3 ) GLOBAL_UNCERTAINTY_ASSIGNED_CONTEXT ( ( #22261 ) ) GLOBAL_UNIT_ASSIGNED_CONTEXT ( ( #4666, #9844, #19025 ) ) REPRESENTATION_CONTEXT ( 'NONE', 'WORKASPACE' ) );
#10509=ORIENTED_EDGE ( 'NONE', *, *, #5991, .F. ) ;
#10517=VECTOR ( 'NONE', #9579, 1000.000000000000000 ) ;
#10527=DIRECTION ( 'NONE',  ( 0.000000000000000000, 0.000000000000000000, 1.000000000000000000 ) ) ;
#10537=EDGE_LOOP ( 'NONE', ( #10428, #4985, #6335, #14734 ) ) ;
#10544=ORIENTED_EDGE ( 'NONE', *, *, #17515, .T. ) ;
#10545=ADVANCED_FACE ( 'NONE', ( #6955 ), #5776, .T. ) ;
#10548=CARTESIAN_POINT ( 'NONE',  ( 0.000000000000000000, 2.999999999999992450, 0.000000000000000000 ) ) ;
#10560=CARTESIAN_POINT ( 'NONE',  ( 37.60054931026104441, 10.94797865062591669, -10.60054931026143166 ) ) ;
#10565=VECTOR ( 'NONE', #9175, 1000.000000000000000 ) ;
#10576=LINE ( 'NONE', #10225, #15961 ) ;
#10597=EDGE_LOOP ( 'NONE', ( #1236, #1005, #6264, #21526 ) ) ;
#10610=AXIS2_PLACEMENT_3D ( 'NONE', #21007, #19116, #1365 ) ;
#10666=VECTOR ( 'NONE', #534, 1000.000000000000000 ) ;
#10696=VECTOR ( 'NONE', #10130, 1000.000000000000000 ) ;
#10700=DIRECTION ( 'NONE',  ( -4.190823558986625216E-31, 1.000000000000000000, -4.190823558986625216E-31 ) ) ;
#10701=LINE ( 'NONE', #18345, #21830 ) ;
#10722=ORIENTED_EDGE ( 'NONE', *, *, #12133, .T. ) ;
#10724=CYLINDRICAL_SURFACE ( 'NONE', #12228, 0.5000000000000017764 ) ;
#10731=DIRECTION ( 'NONE',  ( -1.733449886265891589E-32, 4.190823558986610327E-31, -1.000000000000000000 ) ) ;
#10737=CARTESIAN_POINT ( 'NONE',  ( 2.775557561562891351E-14, 5.500000000000001776, -15.49999999999998579 ) ) ;
#10746=ORIENTED_EDGE ( 'NONE', *, *, #3786, .T. ) ;
#10762=DIRECTION ( 'NONE',  ( -4.190823558986625216E-31, 1.000000000000000000, -4.190823558986625216E-31 ) ) ;
#10777=ORIENTED_EDGE ( 'NONE', *, *, #13484, .T. ) ;
#10779=DIRECTION ( 'NONE',  ( -1.000000000000000000, 4.190823558986610327E-31, -1.733449886265890494E-32 ) ) ;
#10789=CARTESIAN_POINT ( 'NONE',  ( 37.86602540378461157, 11.00000000000000533, -10.86602540378452275 ) ) ;
#10798=EDGE_CURVE ( 'NONE', #2694, #17301, #909, .T. ) ;
#10800=AXIS2_PLACEMENT_3D ( 'NONE', #17142, #6582, #15734 ) ;
#10837=CARTESIAN_POINT ( 'NONE',  ( 37.86602540378462578, -1.973247953923618070E-14, -2.133974596215460817 ) ) ;
#10850=CARTESIAN_POINT ( 'NONE',  ( 42.00000000000014921, 8.000000000000003553, 2.500000000000030198 ) ) ;
#10863=EDGE_CURVE ( 'NONE', #14796, #15246, #1228, .T. ) ;
#10878=CARTESIAN_POINT ( 'NONE',  ( 37.69160037009668685, 10.97664592903650060, -2.482824663591210346 ) ) ;
#10901=CARTESIAN_POINT ( 'NONE',  ( 37.35148779274771158, 0.3618892054749687226, -10.35148779274879693 ) ) ;
#10906=EDGE_LOOP ( 'NONE', ( #18220, #23026, #15132, #1238 ) ) ;
#10910=CARTESIAN_POINT ( 'NONE',  ( 37.18301270189235908, 10.90849364905388263, -10.52451905283837874 ) ) ;
#10931=ORIENTED_EDGE ( 'NONE', *, *, #2006, .F. ) ;
#10940=CARTESIAN_POINT ( 'NONE',  ( 37.04362427881587649, 0.2122202663360489572, -2.545175158706924012 ) ) ;
#10975=AXIS2_PLACEMENT_3D ( 'NONE', #2631, #13216, #4041 ) ;
#10979=CIRCLE ( 'NONE', #13615, 0.5000000000000022204 ) ;
#11022=EDGE_CURVE ( 'NONE', #12892, #16286, #11719, .T. ) ;
#11053=FILL_AREA_STYLE ('',( #20347 ) ) ;
#11064=CARTESIAN_POINT ( 'NONE',  ( 37.36637401601597475, 0.3137297356303543339, -2.633625983984334340 ) ) ;
#11066=DIRECTION ( 'NONE',  ( 0.000000000000000000, 0.000000000000000000, 1.000000000000000000 ) ) ;
#11086=EDGE_CURVE ( 'NONE', #13358, #4671, #10979, .T. ) ;
#11126=CARTESIAN_POINT ( 'NONE',  ( -2.775557561562891351E-14, 10.74999999999998579, -2.566987298107781257 ) ) ;
#11133=ADVANCED_FACE ( 'NONE', ( #1019 ), #12116, .T. ) ;
#11139=PLANE ( 'NONE',  #5512 ) ;
#11144=CYLINDRICAL_SURFACE ( 'NONE', #3656, 0.5000000000000017764 ) ;
#11152=CARTESIAN_POINT ( 'NONE',  ( 42.00000000000012079, 8.000000000000003553, -12.49999999999999645 ) ) ;
#11181=FACE_OUTER_BOUND ( 'NONE', #17062, .T. ) ;
#11189=CARTESIAN_POINT ( 'NONE',  ( 42.50000000000020606, 2.499999999999995115, 5.551115123125782702E-14 ) ) ;
#11192=DIRECTION ( 'NONE',  ( 1.000000000000000000, 3.469446951953611033E-15, 0.000000000000000000 ) ) ;
#11200=DIRECTION ( 'NONE',  ( 1.733449886265891589E-32, -4.190823558986610327E-31, 1.000000000000000000 ) ) ;
#11206=EDGE_LOOP ( 'NONE', ( #14853, #14937, #7734, #5849 ) ) ;
#11231=CARTESIAN_POINT ( 'NONE',  ( 37.43301270189239460, 10.75000000000000178, -2.999999999999959144 ) ) ;
#11239=EDGE_CURVE ( 'NONE', #23201, #7712, #2536, .T. ) ;
#11251=ADVANCED_FACE ( 'NONE', ( #21009 ), #6889, .T. ) ;
#11267=ORIENTED_EDGE ( 'NONE', *, *, #17147, .T. ) ;
#11281=( LENGTH_UNIT ( ) NAMED_UNIT ( * ) SI_UNIT ( .MILLI., .METRE. ) );
#11305=CARTESIAN_POINT ( 'NONE',  ( 37.86602540378466841, 0.000000000000000000, -6.499999999999992006 ) ) ;
#11306=DIRECTION ( 'NONE',  ( -1.000000000000000000, 4.190823558986610327E-31, -1.733449886265890494E-32 ) ) ;
#11358=VECTOR ( 'NONE', #20198, 1000.000000000000000 ) ;
#11365=EDGE_LOOP ( 'NONE', ( #6730, #8382, #20971 ) ) ;
#11373=VECTOR ( 'NONE', #14814, 1000.000000000000000 ) ;
#11377=CARTESIAN_POINT ( 'NONE',  ( 37.86602540378461157, 11.00000000000000000, -10.86602540378450676 ) ) ;
#11387=CARTESIAN_POINT ( 'NONE',  ( 2.775557561562891351E-14, 2.499999999999995115, -12.99999999999999822 ) ) ;
#11395=EDGE_CURVE ( 'NONE', #15946, #18765, #18149, .T. ) ;
#11437=CARTESIAN_POINT ( 'NONE',  ( 5.551115123125782702E-14, 5.499999999999980460, 2.500000000000071498 ) ) ;
#11442=ADVANCED_FACE ( 'NONE', ( #5835 ), #20057, .F. ) ;
#11468=ORIENTED_EDGE ( 'NONE', *, *, #22541, .F. ) ;
#11501=DIRECTION ( 'NONE',  ( 0.000000000000000000, 0.000000000000000000, 1.000000000000000000 ) ) ;
#11503=DIRECTION ( 'NONE',  ( 0.000000000000000000, 0.000000000000000000, -1.000000000000000000 ) ) ;
#11524=CARTESIAN_POINT ( 'NONE',  ( 2.775557561562891351E-14, 10.49999999999998579, -3.000000000000002665 ) ) ;
#11526=CARTESIAN_POINT ( 'NONE',  ( 37.86602540378461157, 0.000000000000000000, -10.86602540378449255 ) ) ;
#11529=TOROIDAL_SURFACE ( 'NONE', #10800, 6.000000000000000888, 3.000000000000000000 ) ;
#11558=CARTESIAN_POINT ( 'NONE',  ( 37.00000000000014211, 10.49999999999999822, -3.000000000000002665 ) ) ;
#11583=VERTEX_POINT ( 'NONE', #1341 ) ;
#11598=CARTESIAN_POINT ( 'NONE',  ( 37.22062532321636752, 0.1155932590976526397, -10.54332536350026750 ) ) ;
#11605=EDGE_LOOP ( 'NONE', ( #15362, #2000, #10544, #7828 ) ) ;
#11651=EDGE_CURVE ( 'NONE', #21020, #7712, #14029, .T. ) ;
#11654=DIRECTION ( 'NONE',  ( -4.190823558986625216E-31, 1.000000000000000000, -4.190823558986625216E-31 ) ) ;
#11655=LINE ( 'NONE', #9908, #7780 ) ;
#11677=CARTESIAN_POINT ( 'NONE',  ( 37.43301270189239460, 0.2500000000000002220, -2.999999999999988898 ) ) ;
#11698=CIRCLE ( 'NONE', #21857, 0.5000000000000004441 ) ;
#11713=DIRECTION ( 'NONE',  ( -1.733449886265891589E-32, 4.190823558986610327E-31, -1.000000000000000000 ) ) ;
#11715=AXIS2_PLACEMENT_3D ( 'NONE', #22249, #4476, #20497 ) ;
#11719=CIRCLE ( 'NONE', #19246, 0.5000000000000000000 ) ;
#11724=CARTESIAN_POINT ( 'NONE',  ( 2.775557561562891351E-14, 0.000000000000000000, -3.000000000000002665 ) ) ;
#11741=CARTESIAN_POINT ( 'NONE',  ( 37.00000000000014211, 0.000000000000000000, -9.999999999999980460 ) ) ;
#11747=( BOUNDED_SURFACE ( )  B_SPLINE_SURFACE ( 3, 2, ( 
 ( #104, #14550, #21407 ),
 ( #7281, #19506, #17980 ),
 ( #8804, #19745, #12435 ),
 ( #3837, #14323, #5399 ),
 ( #12786, #3401, #7047 ),
 ( #14448, #10560, #3510 ),
 ( #3622, #1624, #1734 ),
 ( #19967, #17620, #10789 ) ),
 .UNSPECIFIED., .F., .F., .F. ) 
 B_SPLINE_SURFACE_WITH_KNOTS ( ( 4, 2, 2, 4 ),
 ( 3, 3 ),
 ( 3.665191429188094485, 3.926990816987243171, 4.188790204786392302, 4.712388980384689674 ),
 ( 0.000000000000000000, 1.000000000000000000 ),
 .UNSPECIFIED. ) 
 GEOMETRIC_REPRESENTATION_ITEM ( )  RATIONAL_B_SPLINE_SURFACE ( (
 ( 1.000000000000000000, 0.7905694150421800348, 1.000000000000000000),
 ( 1.000000000000000000, 0.8144940154005646527, 1.000000000000000000),
 ( 1.000000000000000000, 0.8408337562111951602, 1.000000000000000000),
 ( 1.000000000000000000, 0.8912170513578159259, 1.000000000000000000),
 ( 1.000000000000000000, 0.9152160911082961592, 1.000000000000000000),
 ( 1.000000000000000000, 0.9758108578640052322, 1.000000000000000000),
 ( 1.000000000000000000, 1.000509427570091203, 1.000000000000000000),
 ( 1.000000000000000000, 1.000000000000000000, 1.000000000000000000) ) ) 
 REPRESENTATION_ITEM ( '' )  SURFACE ( )  );
#11758=CYLINDRICAL_SURFACE ( 'NONE', #9227, 0.5000000000000004441 ) ;
#11795=CARTESIAN_POINT ( 'NONE',  ( 37.00000000000014211, 0.000000000000000000, -9.999999999999980460 ) ) ;
#11809=AXIS2_PLACEMENT_3D ( 'NONE', #2187, #18420, #7717 ) ;
#11862=FACE_OUTER_BOUND ( 'NONE', #18502, .T. ) ;
#11878=( GEOMETRIC_REPRESENTATION_CONTEXT ( 3 ) GLOBAL_UNCERTAINTY_ASSIGNED_CONTEXT ( ( #6036 ) ) GLOBAL_UNIT_ASSIGNED_CONTEXT ( ( #11281, #9295, #12817 ) ) REPRESENTATION_CONTEXT ( 'NONE', 'WORKASPACE' ) );
#11888=AXIS2_PLACEMENT_3D ( 'NONE', #15610, #2805, #15147 ) ;
#11918=PRODUCT_DEFINITION_CONTEXT ( 'detailed design', #3529, 'design' ) ;
#11920=ORIENTED_EDGE ( 'NONE', *, *, #16191, .T. ) ;
#11925=CIRCLE ( 'NONE', #10057, 0.5000000000000022204 ) ;
#11955=ORIENTED_EDGE ( 'NONE', *, *, #19570, .F. ) ;
#11965=DIRECTION ( 'NONE',  ( 1.000000000000000000, -4.190823558986610327E-31, 1.733449886265890494E-32 ) ) ;
#11972=CARTESIAN_POINT ( 'NONE',  ( 0.000000000000000000, 7.999999999999983125, 0.000000000000000000 ) ) ;
#11996=CARTESIAN_POINT ( 'NONE',  ( 2.775557561562891351E-14, 10.99999999999998579, -3.000000000000002665 ) ) ;
#11997=ADVANCED_FACE ( 'NONE', ( #8089 ), #15606, .F. ) ;
#12028=ADVANCED_FACE ( 'NONE', ( #22795, #18799 ), #20920, .F. ) ;
#12032=ORIENTED_EDGE ( 'NONE', *, *, #14683, .F. ) ;
#12050=PLANE ( 'NONE',  #20062 ) ;
#12060=ORIENTED_EDGE ( 'NONE', *, *, #18463, .T. ) ;
#12067=ADVANCED_FACE ( 'NONE', ( #20811 ), #16897, .T. ) ;
#12114=EDGE_CURVE ( 'NONE', #2883, #3085, #21951, .T. ) ;
#12116=TOROIDAL_SURFACE ( 'NONE', #19636, 6.000000000000000888, 3.000000000000000000 ) ;
#12124=ORIENTED_EDGE ( 'NONE', *, *, #643, .F. ) ;
#12130=EDGE_CURVE ( 'NONE', #17301, #180, #15722, .T. ) ;
#12133=EDGE_CURVE ( 'NONE', #12160, #18765, #5266, .T. ) ;
#12153=ORIENTED_EDGE ( 'NONE', *, *, #19971, .T. ) ;
#12160=VERTEX_POINT ( 'NONE', #10548 ) ;
#12164=EDGE_CURVE ( 'NONE', #17995, #4397, #3390, .T. ) ;
#12182=AXIS2_PLACEMENT_3D ( 'NONE', #9054, #8832, #23191 ) ;
#12209=CIRCLE ( 'NONE', #13730, 6.500000000000023981 ) ;
#12218=CARTESIAN_POINT ( 'NONE',  ( 37.86602540378466841, 0.5000000000000004441, -6.499999999999992006 ) ) ;
#12227=EDGE_CURVE ( 'NONE', #20741, #2357, #7036, .T. ) ;
#12228=AXIS2_PLACEMENT_3D ( 'NONE', #14604, #1890, #11066 ) ;
#12248=VECTOR ( 'NONE', #9399, 1000.000000000000000 ) ;
#12250=CARTESIAN_POINT ( 'NONE',  ( 2.775557561562891351E-14, 2.999999999999992450, -0.4999999999999865663 ) ) ;
#12253=DIRECTION ( 'NONE',  ( 1.733449886265891589E-32, -4.190823558986610327E-31, 1.000000000000000000 ) ) ;
#12264=ORIENTED_EDGE ( 'NONE', *, *, #1455, .F. ) ;
#12291=VECTOR ( 'NONE', #3147, 1000.000000000000000 ) ;
#12321=DIRECTION ( 'NONE',  ( 0.000000000000000000, 0.000000000000000000, -1.000000000000000000 ) ) ;
#12337=ORIENTED_EDGE ( 'NONE', *, *, #23080, .T. ) ;
#12359=ADVANCED_FACE ( 'NONE', ( #18307 ), #9478, .T. ) ;
#12370=DIRECTION ( 'NONE',  ( -1.000000000000000000, 4.190823558986610327E-31, -1.733449886265890494E-32 ) ) ;
#12377=FACE_OUTER_BOUND ( 'NONE', #9923, .T. ) ;
#12393=ORIENTED_EDGE ( 'NONE', *, *, #4021, .T. ) ;
#12420=ORIENTED_EDGE ( 'NONE', *, *, #4398, .T. ) ;
#12426=CARTESIAN_POINT ( 'NONE',  ( 42.00000000000014921, 10.49999999999999822, -0.4999999999999449329 ) ) ;
#12434=DIRECTION ( 'NONE',  ( -1.733449886265891589E-32, 4.190823558986610327E-31, -1.000000000000000000 ) ) ;
#12435=CARTESIAN_POINT ( 'NONE',  ( 37.48161866288229760, 10.82270004028423571, -10.09721192197979711 ) ) ;
#12437=DIRECTION ( 'NONE',  ( -1.733449886265891589E-32, 4.190823558986610327E-31, -1.000000000000000000 ) ) ;
#12438=LINE ( 'NONE', #17985, #3983 ) ;
#12441=CIRCLE ( 'NONE', #14330, 6.000000000000022204 ) ;
#12464=LINE ( 'NONE', #17646, #15327 ) ;
#12480=CARTESIAN_POINT ( 'NONE',  ( 37.00000000000017053, 0.000000000000000000, -6.499999999999964473 ) ) ;
#12487=DIRECTION ( 'NONE',  ( 1.733449886265890494E-32, 4.190823558986611203E-31, -1.000000000000000000 ) ) ;
#12491=AXIS2_PLACEMENT_3D ( 'NONE', #18501, #5924, #16949 ) ;
#12503=TOROIDAL_SURFACE ( 'NONE', #7682, 6.000000000000000000, 0.5000000000000000000 ) ;
#12504=( BOUNDED_CURVE ( )  B_SPLINE_CURVE ( 3, ( #17769, #1658, #7081, #9760 ),
 .UNSPECIFIED., .F., .F. ) 
 B_SPLINE_CURVE_WITH_KNOTS ( ( 4, 4 ),
 ( 1.570796326794896558, 2.617993877991505514 ),
 .UNSPECIFIED. ) 
 CURVE ( )  GEOMETRIC_REPRESENTATION_ITEM ( )  RATIONAL_B_SPLINE_CURVE ( ( 1.000000000000000000, 0.9106836025229571030, 0.9106836025229571030, 1.000000000000000000 ) ) 
 REPRESENTATION_ITEM ( '' )  );
#12527=VECTOR ( 'NONE', #10779, 1000.000000000000000 ) ;
#12528=ORIENTED_EDGE ( 'NONE', *, *, #11086, .T. ) ;
#12541=VERTEX_POINT ( 'NONE', #15109 ) ;
#12572=ORIENTED_EDGE ( 'NONE', *, *, #3481, .F. ) ;
#12579=TOROIDAL_SURFACE ( 'NONE', #2436, 3.500000000000001776, 0.5000000000000000000 ) ;
#12583=CARTESIAN_POINT ( 'NONE',  ( 42.50000000000014921, 8.500000000000003553, -12.49999999999998401 ) ) ;
#12622=ORIENTED_EDGE ( 'NONE', *, *, #4619, .T. ) ;
#12635=DIRECTION ( 'NONE',  ( 0.000000000000000000, 0.000000000000000000, 1.000000000000000000 ) ) ;
#12639=CARTESIAN_POINT ( 'NONE',  ( 2.775557561562891351E-14, 0.000000000000000000, -6.499999999999950262 ) ) ;
#12661=CARTESIAN_POINT ( 'NONE',  ( 42.50000000000014921, 2.999999999999999112, 2.000000000000071054 ) ) ;
#12679=AXIS2_PLACEMENT_3D ( 'NONE', #4972, #12253, #8625 ) ;
#12696=CARTESIAN_POINT ( 'NONE',  ( 2.775557561562891351E-14, 3.000000000000006217, -6.499999999999950262 ) ) ;
#12731=CARTESIAN_POINT ( 'NONE',  ( 37.00000000000006395, 10.75000000000000000, -10.43301270189220276 ) ) ;
#12786=CARTESIAN_POINT ( 'NONE',  ( 37.29045043747289156, 10.91119608832001830, -10.57823792062838386 ) ) ;
#12795=CIRCLE ( 'NONE', #2656, 0.5000000000000022204 ) ;
#12817=( NAMED_UNIT ( * ) SI_UNIT ( $, .STERADIAN. ) SOLID_ANGLE_UNIT ( ) );
#12821=EDGE_CURVE ( 'NONE', #23201, #11583, #17449, .T. ) ;
#12825=ORIENTED_EDGE ( 'NONE', *, *, #643, .T. ) ;
#12846=ADVANCED_FACE ( 'NONE', ( #16952 ), #16730, .F. ) ;
#12862=VERTEX_POINT ( 'NONE', #11558 ) ;
#12879=CARTESIAN_POINT ( 'NONE',  ( 37.51717533640845659, 10.97664592903653791, -2.308399629903466366 ) ) ;
#12880=ORIENTED_EDGE ( 'NONE', *, *, #21677, .T. ) ;
#12892=VERTEX_POINT ( 'NONE', #17308 ) ;
#12898=DIRECTION ( 'NONE',  ( 4.190823558986625216E-31, -1.000000000000000000, 4.190823558986625216E-31 ) ) ;
#12899=DIRECTION ( 'NONE',  ( -4.190823558986625216E-31, 1.000000000000000000, -4.190823558986625216E-31 ) ) ;
#12919=VECTOR ( 'NONE', #19373, 1000.000000000000000 ) ;
#12923=CARTESIAN_POINT ( 'NONE',  ( 37.50000000000014921, 11.00000000000000355, -10.68301270189227559 ) ) ;
#12979=ORIENTED_EDGE ( 'NONE', *, *, #8521, .T. ) ;
#12986=ORIENTED_EDGE ( 'NONE', *, *, #1467, .F. ) ;
#12990=FACE_OUTER_BOUND ( 'NONE', #6977, .T. ) ;
#12996=DIRECTION ( 'NONE',  ( 4.190823558986625216E-31, -1.000000000000000000, 4.190823558986625216E-31 ) ) ;
#12999=DIRECTION ( 'NONE',  ( 3.330669073875454830E-16, 0.000000000000000000, -1.000000000000000000 ) ) ;
#13000=( BOUNDED_SURFACE ( )  B_SPLINE_SURFACE ( 3, 2, ( 
 ( #11231, #21831, #16621 ),
 ( #18408, #21950, #18191 ),
 ( #5842, #7705, #7363 ),
 ( #3937, #9238, #9588 ),
 ( #14526, #539, #16393 ),
 ( #10878, #5718, #12879 ),
 ( #18291, #14878, #18071 ),
 ( #9357, #16508, #5605 ) ),
 .UNSPECIFIED., .F., .F., .T. ) 
 B_SPLINE_SURFACE_WITH_KNOTS ( ( 4, 2, 2, 4 ),
 ( 3, 3 ),
 ( 3.665191429188094929, 3.926990816987243615, 4.188790204786392302, 4.712388980384689674 ),
 ( 0.000000000000000000, 1.000000000000000000 ),
 .UNSPECIFIED. ) 
 GEOMETRIC_REPRESENTATION_ITEM ( )  RATIONAL_B_SPLINE_SURFACE ( (
 ( 1.000000000000000000, 0.7905694150421763711, 1.000000000000000000),
 ( 1.000000000000000000, 0.8144940154005744226, 1.000000000000000000),
 ( 1.000000000000000000, 0.8408337562111710684, 1.000000000000000000),
 ( 1.000000000000000000, 0.8912170513578273612, 1.000000000000000000),
 ( 1.000000000000000000, 0.9152160911082826145, 1.000000000000000000),
 ( 1.000000000000000000, 0.9758108578640108943, 1.000000000000000000),
 ( 1.000000000000000000, 1.000509427570078991, 1.000000000000000000),
 ( 1.000000000000000000, 1.000000000000000000, 1.000000000000000000) ) ) 
 REPRESENTATION_ITEM ( '' )  SURFACE ( )  );
#13005=ORIENTED_EDGE ( 'NONE', *, *, #16204, .T. ) ;
#13017=CARTESIAN_POINT ( 'NONE',  ( 42.50000000000020606, 11.00000000000000000, -12.50000000000001066 ) ) ;
#13043=DIRECTION ( 'NONE',  ( 1.000000000000000000, -1.374679200952743288E-16, -2.095476499216376664E-33 ) ) ;
#13138=CARTESIAN_POINT ( 'NONE',  ( 2.775557561562891351E-14, 0.000000000000000000, -2.133974596215532316 ) ) ;
#13151=FACE_OUTER_BOUND ( 'NONE', #4436, .T. ) ;
#13174=CARTESIAN_POINT ( 'NONE',  ( 2.775557561562891351E-14, 0.000000000000000000, -2.133974596215532316 ) ) ;
#13186=DIRECTION ( 'NONE',  ( -1.000000000000000000, 4.190823558986610327E-31, -1.733449886265890494E-32 ) ) ;
#13205=VERTEX_POINT ( 'NONE', #23070 ) ;
#13215=SPHERICAL_SURFACE ( 'NONE', #2625, 0.5000000000000000000 ) ;
#13216=DIRECTION ( 'NONE',  ( -4.190823558986625216E-31, 1.000000000000000000, -4.190823558986625216E-31 ) ) ;
#13269=DIRECTION ( 'NONE',  ( 1.000000000000000000, -4.437342591868175641E-31, 3.330669073875457788E-16 ) ) ;
#13285=CARTESIAN_POINT ( 'NONE',  ( 42.50000000000014921, 2.999999999999999112, -0.4999999999999726885 ) ) ;
#13310=DIRECTION ( 'NONE',  ( -4.190823558986625216E-31, 1.000000000000000000, -4.190823558986625216E-31 ) ) ;
#13316=CARTESIAN_POINT ( 'NONE',  ( 2.775557561562891351E-14, 0.5000000000000004441, -6.499999999999950262 ) ) ;
#13329=AXIS2_PLACEMENT_3D ( 'NONE', #16382, #7464, #5705 ) ;
#13339=CYLINDRICAL_SURFACE ( 'NONE', #15145, 0.5000000000000004441 ) ;
#13345=DIRECTION ( 'NONE',  ( -4.440892098500626162E-15, 0.000000000000000000, 1.000000000000000000 ) ) ;
#13358=VERTEX_POINT ( 'NONE', #13 ) ;
#13374=CARTESIAN_POINT ( 'NONE',  ( 37.86602540378469683, -6.071532165918824830E-15, -10.86602540378448722 ) ) ;
#13385=DIRECTION ( 'NONE',  ( 4.190823558986621713E-31, 1.000000000000000000, 4.190823558986611203E-31 ) ) ;
#13414=DIRECTION ( 'NONE',  ( 0.000000000000000000, 0.000000000000000000, 1.000000000000000000 ) ) ;
#13429=AXIS2_PLACEMENT_3D ( 'NONE', #11741, #6802, #15502 ) ;
#13466=STYLED_ITEM ( 'NONE', ( #6323 ), #3571 ) ;
#13484=EDGE_CURVE ( 'NONE', #16351, #17191, #16130, .T. ) ;
#13495=CARTESIAN_POINT ( 'NONE',  ( 37.86602540378463999, -6.071532165918824830E-15, -10.86602540378451032 ) ) ;
#13497=LINE ( 'NONE', #20681, #18014 ) ;
#13534=FACE_OUTER_BOUND ( 'NONE', #10906, .T. ) ;
#13560=ORIENTED_EDGE ( 'NONE', *, *, #5799, .F. ) ;
#13565=LINE ( 'NONE', #20749, #4009 ) ;
#13569=EDGE_CURVE ( 'NONE', #18871, #2883, #21438, .T. ) ;
#13609=CARTESIAN_POINT ( 'NONE',  ( 37.51717533640845659, 0.02335407096349230438, -10.69160037009651454 ) ) ;
#13615=AXIS2_PLACEMENT_3D ( 'NONE', #7603, #9257, #21965 ) ;
#13643=AXIS2_PLACEMENT_3D ( 'NONE', #732, #7897, #614 ) ;
#13646=AXIS2_PLACEMENT_3D ( 'NONE', #6885, #23249, #5113 ) ;
#13664=DIRECTION ( 'NONE',  ( -1.000000000000000000, 4.190823558986610327E-31, -1.733449886265890494E-32 ) ) ;
#13666=CYLINDRICAL_SURFACE ( 'NONE', #22432, 0.5000000000000022204 ) ;
#13667=AXIS2_PLACEMENT_3D ( 'NONE', #11152, #21759, #4195 ) ;
#13669=CARTESIAN_POINT ( 'NONE',  ( 37.43301270189239460, 0.2500000000000002220, -9.999999999999953815 ) ) ;
#13677=ORIENTED_EDGE ( 'NONE', *, *, #18281, .T. ) ;
#13699=CIRCLE ( 'NONE', #4231, 0.5000000000000017764 ) ;
#13703=VERTEX_POINT ( 'NONE', #23003 ) ;
#13709=ORIENTED_EDGE ( 'NONE', *, *, #23182, .T. ) ;
#13730=AXIS2_PLACEMENT_3D ( 'NONE', #17278, #14940, #15171 ) ;
#13731=CARTESIAN_POINT ( 'NONE',  ( 2.775557561562891351E-14, 8.000000000000003553, -15.49999999999998579 ) ) ;
#13736=ORIENTED_EDGE ( 'NONE', *, *, #591, .T. ) ;
#13739=VERTEX_POINT ( 'NONE', #7579 ) ;
#13743=CARTESIAN_POINT ( 'NONE',  ( 42.50000000000020606, 10.49999999999999822, -12.50000000000001066 ) ) ;
#13762=VERTEX_POINT ( 'NONE', #18510 ) ;
#13783=EDGE_CURVE ( 'NONE', #13762, #16689, #21941, .T. ) ;
#13792=LINE ( 'NONE', #2975, #19712 ) ;
#13797=CIRCLE ( 'NONE', #7802, 0.5000000000000018874 ) ;
#13836=CARTESIAN_POINT ( 'NONE',  ( 37.69160037009659447, 0.02335407096354361403, -10.51717533640881364 ) ) ;
#13841=CARTESIAN_POINT ( 'NONE',  ( 2.775557561562891351E-14, -1.387778780781445676E-14, -12.50000000000001066 ) ) ;
#13848=( GEOMETRIC_REPRESENTATION_CONTEXT ( 3 ) GLOBAL_UNCERTAINTY_ASSIGNED_CONTEXT ( ( #19927 ) ) GLOBAL_UNIT_ASSIGNED_CONTEXT ( ( #16888, #4424, #10081 ) ) REPRESENTATION_CONTEXT ( 'NONE', 'WORKASPACE' ) );
#13861=ADVANCED_FACE ( 'NONE', ( #15435 ), #13215, .F. ) ;
#13862=LINE ( 'NONE', #9033, #15959 ) ;
#13884=DIRECTION ( 'NONE',  ( 4.190823558986626092E-31, -1.000000000000000000, -4.190823558986610327E-31 ) ) ;
#13888=LINE ( 'NONE', #19293, #10696 ) ;
#13922=CIRCLE ( 'NONE', #3773, 4.366025403784456138 ) ;
#13977=ORIENTED_EDGE ( 'NONE', *, *, #16191, .F. ) ;
#14004=DIRECTION ( 'NONE',  ( -1.000000000000000000, 4.190823558986610327E-31, -1.733449886265890494E-32 ) ) ;
#14013=TOROIDAL_SURFACE ( 'NONE', #872, 2.500000000000000000, 0.5000000000000000000 ) ;
#14029=CIRCLE ( 'NONE', #14783, 0.5000000000000015543 ) ;
#14045=AXIS2_PLACEMENT_3D ( 'NONE', #7703, #12996, #13345 ) ;
#14057=DIRECTION ( 'NONE',  ( -1.000000000000000000, 4.190823558986610327E-31, -1.733449886265890494E-32 ) ) ;
#14101=ORIENTED_EDGE ( 'NONE', *, *, #7690, .T. ) ;
#14106=ADVANCED_FACE ( 'NONE', ( #21224 ), #19430, .F. ) ;
#14113=LINE ( 'NONE', #21297, #19364 ) ;
#14177=CARTESIAN_POINT ( 'NONE',  ( 0.000000000000000000, 11.00000000000000000, -10.86602540378443749 ) ) ;
#14185=CARTESIAN_POINT ( 'NONE',  ( 2.775557561562891351E-14, 10.99999999999998579, -3.000000000000002665 ) ) ;
#14200=EDGE_LOOP ( 'NONE', ( #9592, #20278, #18413, #3051 ) ) ;
#14203=PRODUCT ( 'Handle Clip', 'Handle Clip', '', ( #14697 ) ) ;
#14262=DIRECTION ( 'NONE',  ( -1.733449886265891589E-32, 4.190823558986610327E-31, -1.000000000000000000 ) ) ;
#14300=EDGE_CURVE ( 'NONE', #2718, #15424, #12795, .T. ) ;
#14323=CARTESIAN_POINT ( 'NONE',  ( 37.42127086598691221, 10.78233971064650198, -10.42127086598680741 ) ) ;
#14330=AXIS2_PLACEMENT_3D ( 'NONE', #1759, #17139, #15259 ) ;
#14352=CIRCLE ( 'NONE', #842, 0.5000000000000017764 ) ;
#14357=AXIS2_PLACEMENT_3D ( 'NONE', #8911, #5269, #16182 ) ;
#14361=AXIS2_PLACEMENT_3D ( 'NONE', #1390, #21156, #23038 ) ;
#14374=CARTESIAN_POINT ( 'NONE',  ( 2.775557561562891351E-14, 2.499999999999998668, -6.499999999999950262 ) ) ;
#14376=CIRCLE ( 'NONE', #10975, 0.5000000000000022204 ) ;
#14391=ORIENTED_EDGE ( 'NONE', *, *, #14656, .F. ) ;
#14448=CARTESIAN_POINT ( 'NONE',  ( 37.51717533640845659, 10.97664592903658232, -10.69160037009666020 ) ) ;
#14450=CARTESIAN_POINT ( 'NONE',  ( 2.775557561562891351E-14, 2.999999999999999112, -12.99999999999999822 ) ) ;
#14455=AXIS2_PLACEMENT_3D ( 'NONE', #6139, #9319, #20024 ) ;
#14458=AXIS2_PLACEMENT_3D ( 'NONE', #22270, #2856, #637 ) ;
#14526=CARTESIAN_POINT ( 'NONE',  ( 37.57823792062858104, 10.91119608832008581, -2.709549562527672872 ) ) ;
#14529=CARTESIAN_POINT ( 'NONE',  ( 2.775557561562891351E-14, 8.000000000000003553, -15.49999999999998579 ) ) ;
#14550=CARTESIAN_POINT ( 'NONE',  ( 37.34641016151397963, 10.60000000000007425, -10.34641016151376824 ) ) ;
#14557=CARTESIAN_POINT ( 'NONE',  ( 37.00000000000014211, 11.00000000000000000, -3.000000000000002665 ) ) ;
#14558=EDGE_CURVE ( 'NONE', #13358, #19695, #4158, .T. ) ;
#14567=ADVANCED_FACE ( 'NONE', ( #5063 ), #8708, .T. ) ;
#14576=VERTEX_POINT ( 'NONE', #5534 ) ;
#14584=FACE_OUTER_BOUND ( 'NONE', #16173, .T. ) ;
#14586=EDGE_CURVE ( 'NONE', #4671, #17191, #13922, .T. ) ;
#14604=CARTESIAN_POINT ( 'NONE',  ( 2.775557561562891351E-14, 10.49999999999998579, -2.133974596215532316 ) ) ;
#14612=CIRCLE ( 'NONE', #10115, 2.500000000000009326 ) ;
#14622=EDGE_LOOP ( 'NONE', ( #1322, #16975, #19250 ) ) ;
#14638=PRODUCT_DEFINITION_FORMATION_WITH_SPECIFIED_SOURCE ( 'ANY', '', #14203, .NOT_KNOWN. ) ;
#14656=EDGE_CURVE ( 'NONE', #13358, #18075, #10701, .T. ) ;
#14660=DIRECTION ( 'NONE',  ( 1.374679200952786429E-16, -1.000000000000000000, 0.000000000000000000 ) ) ;
#14669=DIRECTION ( 'NONE',  ( -1.000000000000000000, 4.190823558986611203E-31, 1.733449886265891589E-32 ) ) ;
#14683=EDGE_CURVE ( 'NONE', #4498, #16351, #1985, .T. ) ;
#14697=PRODUCT_CONTEXT ( 'NONE', #3962, 'mechanical' ) ;
#14704=CARTESIAN_POINT ( 'NONE',  ( 2.775557561562891351E-14, 0.5000000000000108802, -9.999999999999968026 ) ) ;
#14711=EDGE_CURVE ( 'NONE', #180, #15946, #12441, .T. ) ;
#14734=ORIENTED_EDGE ( 'NONE', *, *, #594, .F. ) ;
#14750=CARTESIAN_POINT ( 'NONE',  ( 2.775557561562891351E-14, 7.999999999999983125, -0.4999999999999865663 ) ) ;
#14783=AXIS2_PLACEMENT_3D ( 'NONE', #6622, #15665, #5094 ) ;
#14792=CARTESIAN_POINT ( 'NONE',  ( 2.775557561562891351E-14, 0.000000000000000000, -0.4999999999999865663 ) ) ;
#14795=CIRCLE ( 'NONE', #20080, 3.500000000000013323 ) ;
#14796=VERTEX_POINT ( 'NONE', #2453 ) ;
#14797=AXIS2_PLACEMENT_3D ( 'NONE', #6334, #13385, #8323 ) ;
#14805=DIRECTION ( 'NONE',  ( -1.756300210255732376E-61, 4.190823558986625216E-31, 1.000000000000000000 ) ) ;
#14808=LINE ( 'NONE', #11387, #3874 ) ;
#14810=AXIS2_PLACEMENT_3D ( 'NONE', #19205, #20981, #4618 ) ;
#14814=DIRECTION ( 'NONE',  ( -1.000000000000000000, 4.190823558986610327E-31, -1.733449886265890494E-32 ) ) ;
#14829=CARTESIAN_POINT ( 'NONE',  ( 2.775557561562891351E-14, 2.499999999999995115, -12.99999999999999822 ) ) ;
#14836=LINE ( 'NONE', #11189, #19421 ) ;
#14837=ADVANCED_FACE ( 'NONE', ( #6227 ), #18575, .T. ) ;
#14841=DIRECTION ( 'NONE',  ( 4.190823558986625216E-31, -1.000000000000000000, 4.190823558986625216E-31 ) ) ;
#14853=ORIENTED_EDGE ( 'NONE', *, *, #7340, .F. ) ;
#14870=DIRECTION ( 'NONE',  ( 1.000000000000000000, -4.190823558986610327E-31, 1.733449886265890494E-32 ) ) ;
#14877=EDGE_CURVE ( 'NONE', #3943, #7856, #1926, .T. ) ;
#14878=CARTESIAN_POINT ( 'NONE',  ( 37.73505106183078794, 10.99999999999229239, -2.264948938166786441 ) ) ;
#14909=DIRECTION ( 'NONE',  ( -1.733449886265891589E-32, 4.190823558986610327E-31, -1.000000000000000000 ) ) ;
#14937=ORIENTED_EDGE ( 'NONE', *, *, #14711, .T. ) ;
#14940=DIRECTION ( 'NONE',  ( 4.190823558986625216E-31, -1.000000000000000000, 4.190823558986625216E-31 ) ) ;
#14944=DIRECTION ( 'NONE',  ( 0.000000000000000000, 0.000000000000000000, 1.000000000000000000 ) ) ;
#14955=TOROIDAL_SURFACE ( 'NONE', #4816, 6.000000000000000000, 0.5000000000000000000 ) ;
#14956=CARTESIAN_POINT ( 'NONE',  ( 42.00000000000012079, 8.000000000000003553, -12.49999999999999645 ) ) ;
#15015=FACE_OUTER_BOUND ( 'NONE', #1965, .T. ) ;
#15036=DIRECTION ( 'NONE',  ( 0.000000000000000000, 0.5000000000000026645, 0.8660254037844372643 ) ) ;
#15040=VERTEX_POINT ( 'NONE', #7043 ) ;
#15060=FACE_BOUND ( 'NONE', #3687, .T. ) ;
#15070=EDGE_LOOP ( 'NONE', ( #2589, #513, #12528, #2181 ) ) ;
#15078=CARTESIAN_POINT ( 'NONE',  ( 37.00000000000014211, 11.00000000000000000, -3.000000000000002665 ) ) ;
#15109=CARTESIAN_POINT ( 'NONE',  ( 37.00000000000014211, 0.5000000000000004441, -3.000000000000002665 ) ) ;
#15132=ORIENTED_EDGE ( 'NONE', *, *, #21956, .T. ) ;
#15140=DIRECTION ( 'NONE',  ( 3.330669073875454830E-16, 0.000000000000000000, -1.000000000000000000 ) ) ;
#15145=AXIS2_PLACEMENT_3D ( 'NONE', #7921, #8589, #20287 ) ;
#15147=DIRECTION ( 'NONE',  ( -1.733449886265891589E-32, 4.190823558986610327E-31, -1.000000000000000000 ) ) ;
#15155=LINE ( 'NONE', #4449, #2449 ) ;
#15159=LINE ( 'NONE', #22462, #16042 ) ;
#15171=DIRECTION ( 'NONE',  ( -4.440892098500626162E-15, 0.000000000000000000, 1.000000000000000000 ) ) ;
#15187=ADVANCED_FACE ( 'NONE', ( #22077 ), #22606, .T. ) ;
#15190=VERTEX_POINT ( 'NONE', #2193 ) ;
#15236=ORIENTED_EDGE ( 'NONE', *, *, #18281, .F. ) ;
#15240=LINE ( 'NONE', #13731, #12291 ) ;
#15246=VERTEX_POINT ( 'NONE', #4765 ) ;
#15257=CARTESIAN_POINT ( 'NONE',  ( 42.50000000000014921, 8.000000000000003553, -12.49999999999998401 ) ) ;
#15259=DIRECTION ( 'NONE',  ( 0.000000000000000000, 0.000000000000000000, 1.000000000000000000 ) ) ;
#15305=CIRCLE ( 'NONE', #3359, 0.5000000000000017764 ) ;
#15310=ORIENTED_EDGE ( 'NONE', *, *, #8521, .F. ) ;
#15327=VECTOR ( 'NONE', #1764, 1000.000000000000000 ) ;
#15328=CARTESIAN_POINT ( 'NONE',  ( 42.50000000000014921, 0.5000000000000004441, -12.49999999999998401 ) ) ;
#15331=EDGE_CURVE ( 'NONE', #8906, #22878, #2130, .T. ) ;
#15332=FACE_OUTER_BOUND ( 'NONE', #3388, .T. ) ;
#15341=ORIENTED_EDGE ( 'NONE', *, *, #2006, .T. ) ;
#15362=ORIENTED_EDGE ( 'NONE', *, *, #12133, .F. ) ;
#15369=ORIENTED_EDGE ( 'NONE', *, *, #18026, .T. ) ;
#15370=ORIENTED_EDGE ( 'NONE', *, *, #6771, .T. ) ;
#15389=DIRECTION ( 'NONE',  ( -1.000000000000000000, 4.190823558986610327E-31, -1.733449886265890494E-32 ) ) ;
#15395=EDGE_CURVE ( 'NONE', #1098, #16034, #90, .T. ) ;
#15419=EDGE_LOOP ( 'NONE', ( #5467, #17820, #10509, #20859 ) ) ;
#15424=VERTEX_POINT ( 'NONE', #18144 ) ;
#15435=FACE_OUTER_BOUND ( 'NONE', #23056, .T. ) ;
#15455=EDGE_CURVE ( 'NONE', #6443, #13762, #2696, .T. ) ;
#15482=ORIENTED_EDGE ( 'NONE', *, *, #22210, .T. ) ;
#15484=PRODUCT_DEFINITION_SHAPE ( 'NONE', 'NONE',  #18401 ) ;
#15502=DIRECTION ( 'NONE',  ( 0.000000000000000000, 4.190823558986606824E-31, -1.000000000000000000 ) ) ;
#15506=CARTESIAN_POINT ( 'NONE',  ( 42.50000000000014921, 2.499999999999998668, -12.49999999999998401 ) ) ;
#15520=DIRECTION ( 'NONE',  ( -1.733449886265891589E-32, 4.190823558986610327E-31, -1.000000000000000000 ) ) ;
#15530=FACE_OUTER_BOUND ( 'NONE', #16515, .T. ) ;
#15538=ADVANCED_FACE ( 'NONE', ( #966 ), #2708, .T. ) ;
#15548=FACE_OUTER_BOUND ( 'NONE', #4248, .T. ) ;
#15588=EDGE_CURVE ( 'NONE', #16689, #12862, #11698, .T. ) ;
#15606=SPHERICAL_SURFACE ( 'NONE', #14797, 0.5000000000000000000 ) ;
#15610=CARTESIAN_POINT ( 'NONE',  ( 2.775557561562891351E-14, 10.49999999999999822, -6.499999999999950262 ) ) ;
#15616=DIRECTION ( 'NONE',  ( 4.190823558986625216E-31, -1.000000000000000000, 4.190823558986625216E-31 ) ) ;
#15628=ORIENTED_EDGE ( 'NONE', *, *, #5918, .T. ) ;
#15652=ORIENTED_EDGE ( 'NONE', *, *, #15832, .F. ) ;
#15665=DIRECTION ( 'NONE',  ( -0.4472135954999586493, 0.7745966692414837373, -0.4472135954999567065 ) ) ;
#15678=ORIENTED_EDGE ( 'NONE', *, *, #393, .T. ) ;
#15699=COLOUR_RGB ( '', 0.40784314, 0.44705882, 0.49803922) ;
#15706=ORIENTED_EDGE ( 'NONE', *, *, #55, .F. ) ;
#15719=ORIENTED_EDGE ( 'NONE', *, *, #5799, .T. ) ;
#15722=LINE ( 'NONE', #15949, #12527 ) ;
#15734=DIRECTION ( 'NONE',  ( -1.756300210255732376E-61, 4.190823558986625216E-31, 1.000000000000000000 ) ) ;
#15770=ORIENTED_EDGE ( 'NONE', *, *, #6940, .F. ) ;
#15818=CARTESIAN_POINT ( 'NONE',  ( 37.00000000000017053, 0.5000000000000004441, -6.499999999999964473 ) ) ;
#15822=ORIENTED_EDGE ( 'NONE', *, *, #21293, .T. ) ;
#15832=EDGE_CURVE ( 'NONE', #22878, #23201, #5713, .T. ) ;
#15840=CARTESIAN_POINT ( 'NONE',  ( 42.00000000000020606, 2.999999999999999112, -15.50000000000004086 ) ) ;
#15863=DIRECTION ( 'NONE',  ( 1.000000000000000000, 0.000000000000000000, 0.000000000000000000 ) ) ;
#15874=ORIENTED_EDGE ( 'NONE', *, *, #3924, .T. ) ;
#15879=VERTEX_POINT ( 'NONE', #9628 ) ;
#15920=ORIENTED_EDGE ( 'NONE', *, *, #14300, .T. ) ;
#15941=ORIENTED_EDGE ( 'NONE', *, *, #15331, .T. ) ;
#15946=VERTEX_POINT ( 'NONE', #698 ) ;
#15949=CARTESIAN_POINT ( 'NONE',  ( 2.775557561562891351E-14, 8.500000000000003553, -12.50000000000001066 ) ) ;
#15952=CARTESIAN_POINT ( 'NONE',  ( 42.00000000000014921, 5.500000000000001776, -15.00000000000001421 ) ) ;
#15959=VECTOR ( 'NONE', #12434, 1000.000000000000000 ) ;
#15961=VECTOR ( 'NONE', #1302, 1000.000000000000000 ) ;
#15963=CYLINDRICAL_SURFACE ( 'NONE', #2141, 0.5000000000000004441 ) ;
#15987=DIRECTION ( 'NONE',  ( -1.000000000000000000, 4.190823558986610327E-31, -1.733449886265890494E-32 ) ) ;
#15990=DIRECTION ( 'NONE',  ( -1.756300210255732376E-61, 4.190823558986625216E-31, 1.000000000000000000 ) ) ;
#16018=CARTESIAN_POINT ( 'NONE',  ( 2.775557561562891351E-14, 2.999999999999992450, -0.4999999999999865663 ) ) ;
#16020=DIRECTION ( 'NONE',  ( 1.000000000000000000, 0.000000000000000000, 0.000000000000000000 ) ) ;
#16030=ORIENTED_EDGE ( 'NONE', *, *, #23196, .T. ) ;
#16034=VERTEX_POINT ( 'NONE', #6683 ) ;
#16042=VECTOR ( 'NONE', #20702, 1000.000000000000000 ) ;
#16069=CARTESIAN_POINT ( 'NONE',  ( 42.50000000000014921, 2.999999999999999112, -12.49999999999998401 ) ) ;
#16130=CIRCLE ( 'NONE', #5627, 0.5000000000000004441 ) ;
#16132=CYLINDRICAL_SURFACE ( 'NONE', #18481, 0.5000000000000017764 ) ;
#16142=EDGE_LOOP ( 'NONE', ( #6626, #22033, #16170, #15678 ) ) ;
#16170=ORIENTED_EDGE ( 'NONE', *, *, #1071, .F. ) ;
#16171=ORIENTED_EDGE ( 'NONE', *, *, #10863, .F. ) ;
#16172=ADVANCED_FACE ( 'NONE', ( #1727 ), #3952, .T. ) ;
#16173=EDGE_LOOP ( 'NONE', ( #9652, #13005, #6820, #2524 ) ) ;
#16182=DIRECTION ( 'NONE',  ( 0.000000000000000000, 0.000000000000000000, 1.000000000000000000 ) ) ;
#16191=EDGE_CURVE ( 'NONE', #16369, #11583, #21288, .T. ) ;
#16204=EDGE_CURVE ( 'NONE', #4397, #6390, #3824, .T. ) ;
#16227=EDGE_LOOP ( 'NONE', ( #12060, #19753, #4529, #6707 ) ) ;
#16230=CARTESIAN_POINT ( 'NONE',  ( 37.45482484129320966, 0.2122202663359486485, -2.956375721184415717 ) ) ;
#16241=VECTOR ( 'NONE', #2045, 1000.000000000000000 ) ;
#16253=ORIENTED_EDGE ( 'NONE', *, *, #18209, .F. ) ;
#16286=VERTEX_POINT ( 'NONE', #13138 ) ;
#16306=CARTESIAN_POINT ( 'NONE',  ( 37.00000000000017053, 0.2500000000000002220, -10.43301270189217433 ) ) ;
#16316=CARTESIAN_POINT ( 'NONE',  ( 37.48161866288228339, 0.1772999597157746965, -10.09721192197987705 ) ) ;
#16324=FACE_OUTER_BOUND ( 'NONE', #20918, .T. ) ;
#16346=AXIS2_PLACEMENT_3D ( 'NONE', #8939, #11, #18001 ) ;
#16351=VERTEX_POINT ( 'NONE', #11126 ) ;
#16353=CARTESIAN_POINT ( 'NONE',  ( 37.46001462128806736, 0.1698019261547118741, -2.539985378711791419 ) ) ;
#16363=FACE_OUTER_BOUND ( 'NONE', #16227, .T. ) ;
#16369=VERTEX_POINT ( 'NONE', #20200 ) ;
#16373=EDGE_LOOP ( 'NONE', ( #3056, #18775, #5012, #5960 ) ) ;
#16380=ORIENTED_EDGE ( 'NONE', *, *, #2463, .T. ) ;
#16382=CARTESIAN_POINT ( 'NONE',  ( 37.00000000000014211, 0.000000000000000000, -9.999999999999980460 ) ) ;
#16393=CARTESIAN_POINT ( 'NONE',  ( 37.29045043747289156, 10.91119608832006449, -2.421762079371571730 ) ) ;
#16404=ORIENTED_EDGE ( 'NONE', *, *, #13783, .T. ) ;
#16409=DIRECTION ( 'NONE',  ( 0.000000000000000000, 0.000000000000000000, 1.000000000000000000 ) ) ;
#16423=FACE_OUTER_BOUND ( 'NONE', #10079, .T. ) ;
#16429=ADVANCED_FACE ( 'NONE', ( #4532 ), #19352, .F. ) ;
#16454=MECHANICAL_DESIGN_GEOMETRIC_PRESENTATION_REPRESENTATION('',(#13466),#10475);
#16458=AXIS2_PLACEMENT_3D ( 'NONE', #4566, #15389, #22577 ) ;
#16462=ORIENTED_EDGE ( 'NONE', *, *, #896, .F. ) ;
#16468=DIRECTION ( 'NONE',  ( 1.000000000000000000, -4.190823558986610327E-31, 1.733449886265890494E-32 ) ) ;
#16469=CARTESIAN_POINT ( 'NONE',  ( 37.51717533640922397, 0.02335407096342949698, -2.308399629903371331 ) ) ;
#16478=CARTESIAN_POINT ( 'NONE',  ( 2.775557561562891351E-14, 0.5000000000000108802, -9.999999999999968026 ) ) ;
#16508=CARTESIAN_POINT ( 'NONE',  ( 37.86602540378468262, 11.00000000000000533, -2.133974596215522990 ) ) ;
#16515=EDGE_LOOP ( 'NONE', ( #10165, #19628, #12032, #19170 ) ) ;
#16522=EDGE_CURVE ( 'NONE', #13703, #4671, #288, .T. ) ;
#16526=CARTESIAN_POINT ( 'NONE',  ( 42.00000000000020606, 2.999999999999999112, -0.4999999999999449329 ) ) ;
#16534=CARTESIAN_POINT ( 'NONE',  ( 42.50000000000017764, 5.500000000000001776, 2.500000000000071498 ) ) ;
#16544=( BOUNDED_CURVE ( )  B_SPLINE_CURVE ( 3, ( #7249, #17704, #23012, #5000 ),
 .UNSPECIFIED., .F., .F. ) 
 B_SPLINE_CURVE_WITH_KNOTS ( ( 4, 4 ),
 ( 3.665191429188049632, 4.712388980384689674 ),
 .UNSPECIFIED. ) 
 CURVE ( )  GEOMETRIC_REPRESENTATION_ITEM ( )  RATIONAL_B_SPLINE_CURVE ( ( 1.000000000000000000, 0.9106836025229521070, 0.9106836025229521070, 1.000000000000000000 ) ) 
 REPRESENTATION_ITEM ( '' )  );
#16620=CARTESIAN_POINT ( 'NONE',  ( 0.000000000000000000, 0.5000000000000108802, -10.86602540378443749 ) ) ;
#16621=CARTESIAN_POINT ( 'NONE',  ( 37.00000000000030553, 10.74999999999999822, -2.566987298107756388 ) ) ;
#16643=CIRCLE ( 'NONE', #4633, 2.500000000000008882 ) ;
#16689=VERTEX_POINT ( 'NONE', #871 ) ;
#16694=CARTESIAN_POINT ( 'NONE',  ( 37.73505106183394986, 7.718611010957700083E-12, -2.264948938170268544 ) ) ;
#16700=DIRECTION ( 'NONE',  ( -4.190823558986625216E-31, 1.000000000000000000, -4.190823558986625216E-31 ) ) ;
#16706=EDGE_CURVE ( 'NONE', #7197, #18871, #14376, .T. ) ;
#16711=DIRECTION ( 'NONE',  ( -1.000000000000000000, 4.190823558986610327E-31, -1.733449886265890494E-32 ) ) ;
#16730=CYLINDRICAL_SURFACE ( 'NONE', #14458, 0.5000000000000022204 ) ;
#16751=CIRCLE ( 'NONE', #3267, 2.500000000000008882 ) ;
#16773=DIRECTION ( 'NONE',  ( 0.000000000000000000, -4.190823558986610327E-31, 1.000000000000000000 ) ) ;
#16784=DIRECTION ( 'NONE',  ( -4.190823558986625216E-31, 1.000000000000000000, -4.190823558986625216E-31 ) ) ;
#16820=AXIS2_PLACEMENT_3D ( 'NONE', #6004, #2575, #7642 ) ;
#16863=EDGE_LOOP ( 'NONE', ( #14391, #20072, #892, #2030 ) ) ;
#16888=( LENGTH_UNIT ( ) NAMED_UNIT ( * ) SI_UNIT ( .MILLI., .METRE. ) );
#16897=CYLINDRICAL_SURFACE ( 'NONE', #17038, 0.5000000000000022204 ) ;
#16908=DIRECTION ( 'NONE',  ( 4.190823558986625216E-31, -1.000000000000000000, 4.190823558986625216E-31 ) ) ;
#16911=CARTESIAN_POINT ( 'NONE',  ( 2.775557561562891351E-14, 1.387778780781445676E-14, -9.999999999999968026 ) ) ;
#16938=ORIENTED_EDGE ( 'NONE', *, *, #16522, .F. ) ;
#16949=DIRECTION ( 'NONE',  ( 0.000000000000000000, 0.000000000000000000, -1.000000000000000000 ) ) ;
#16952=FACE_OUTER_BOUND ( 'NONE', #7098, .T. ) ;
#16955=CARTESIAN_POINT ( 'NONE',  ( 2.775557561562891351E-14, 0.5000000000000004441, -6.499999999999950262 ) ) ;
#16971=EDGE_CURVE ( 'NONE', #14796, #17995, #9143, .T. ) ;
#16975=ORIENTED_EDGE ( 'NONE', *, *, #22353, .T. ) ;
#16977=ORIENTED_EDGE ( 'NONE', *, *, #18805, .F. ) ;
#17017=AXIS2_PLACEMENT_3D ( 'NONE', #15078, #640, #4930 ) ;
#17035=VECTOR ( 'NONE', #17553, 1000.000000000000000 ) ;
#17036=AXIS2_PLACEMENT_3D ( 'NONE', #15257, #11965, #22451 ) ;
#17038=AXIS2_PLACEMENT_3D ( 'NONE', #7973, #13269, #15140 ) ;
#17045=DIRECTION ( 'NONE',  ( 1.000000000000000000, -4.190823558986610327E-31, 1.733449886265890494E-32 ) ) ;
#17057=DIRECTION ( 'NONE',  ( 0.000000000000000000, 0.000000000000000000, 1.000000000000000000 ) ) ;
#17060=DIRECTION ( 'NONE',  ( -1.000000000000000000, 4.190823558986610327E-31, -1.733449886265890494E-32 ) ) ;
#17062=EDGE_LOOP ( 'NONE', ( #9062, #15719, #15369, #12264 ) ) ;
#17081=CIRCLE ( 'NONE', #6974, 3.000000000000011546 ) ;
#17116=CARTESIAN_POINT ( 'NONE',  ( 37.86602540378474657, -6.071532165918824830E-15, -10.86602540378446058 ) ) ;
#17122=ORIENTED_EDGE ( 'NONE', *, *, #18026, .F. ) ;
#17124=CIRCLE ( 'NONE', #7015, 0.5000000000000022204 ) ;
#17139=DIRECTION ( 'NONE',  ( -4.190823558986625216E-31, 1.000000000000000000, -4.190823558986625216E-31 ) ) ;
#17142=CARTESIAN_POINT ( 'NONE',  ( 2.775557561562891351E-14, 3.000000000000006217, -6.499999999999950262 ) ) ;
#17147=EDGE_CURVE ( 'NONE', #23201, #16369, #8364, .T. ) ;
#17159=ORIENTED_EDGE ( 'NONE', *, *, #12227, .T. ) ;
#17167=CARTESIAN_POINT ( 'NONE',  ( 2.775557561562891351E-14, 10.99999999999998579, -2.133974596215532316 ) ) ;
#17175=DIRECTION ( 'NONE',  ( 0.000000000000000000, 0.000000000000000000, 1.000000000000000000 ) ) ;
#17179=AXIS2_PLACEMENT_3D ( 'NONE', #3536, #5295, #5648 ) ;
#17191=VERTEX_POINT ( 'NONE', #17167 ) ;
#17221=ORIENTED_EDGE ( 'NONE', *, *, #14300, .F. ) ;
#17226=VERTEX_POINT ( 'NONE', #18955 ) ;
#17230=CARTESIAN_POINT ( 'NONE',  ( 2.775557561562891351E-14, 8.000000000000003553, -6.499999999999950262 ) ) ;
#17259=DIRECTION ( 'NONE',  ( -1.000000000000000000, 4.190823558986610327E-31, -1.733449886265890494E-32 ) ) ;
#17278=CARTESIAN_POINT ( 'NONE',  ( 2.775557561562891351E-14, 2.999999999999999112, -6.499999999999950262 ) ) ;
#17301=VERTEX_POINT ( 'NONE', #12583 ) ;
#17303=AXIS2_PLACEMENT_3D ( 'NONE', #1416, #4712, #21192 ) ;
#17308=CARTESIAN_POINT ( 'NONE',  ( 5.551115123125782702E-14, 0.2500000000000002220, -2.566987298107781257 ) ) ;
#17324=ORIENTED_EDGE ( 'NONE', *, *, #9390, .T. ) ;
#17327=EDGE_LOOP ( 'NONE', ( #20183, #6150, #21445, #518 ) ) ;
#17353=FILL_AREA_STYLE_COLOUR ( '', #15699 ) ;
#17367=CARTESIAN_POINT ( 'NONE',  ( 42.50000000000014921, 0.000000000000000000, -12.49999999999998401 ) ) ;
#17400=CARTESIAN_POINT ( 'NONE',  ( 37.52451905283849953, 0.09150635094611496434, -10.18301270189224539 ) ) ;
#17408=AXIS2_PLACEMENT_3D ( 'NONE', #19493, #10437, #5385 ) ;
#17418=ORIENTED_EDGE ( 'NONE', *, *, #20471, .F. ) ;
#17430=DIRECTION ( 'NONE',  ( 1.000000000000000000, -4.190823558986610327E-31, 1.733449886265890494E-32 ) ) ;
#17449=CIRCLE ( 'NONE', #13329, 0.5000000000000009992 ) ;
#17486=DIRECTION ( 'NONE',  ( 4.190823558986625216E-31, -1.000000000000000000, 4.190823558986625216E-31 ) ) ;
#17515=EDGE_CURVE ( 'NONE', #6309, #5339, #14808, .T. ) ;
#17538=ORIENTED_EDGE ( 'NONE', *, *, #14683, .T. ) ;
#17543=DIRECTION ( 'NONE',  ( 1.000000000000000000, 2.664535259100391869E-15, 0.000000000000000000 ) ) ;
#17544=DIRECTION ( 'NONE',  ( 1.000000000000000000, -4.190823558986610327E-31, 1.733449886265890494E-32 ) ) ;
#17553=DIRECTION ( 'NONE',  ( 1.000000000000000000, -4.190823558986610327E-31, 1.733449886265890494E-32 ) ) ;
#17563=ORIENTED_EDGE ( 'NONE', *, *, #594, .T. ) ;
#17604=EDGE_CURVE ( 'NONE', #2357, #15246, #16643, .T. ) ;
#17620=CARTESIAN_POINT ( 'NONE',  ( 37.86602540378468262, 11.00000000000000533, -10.86602540378449255 ) ) ;
#17623=DIRECTION ( 'NONE',  ( -1.000000000000000000, 4.190823558986610327E-31, -1.733449886265890494E-32 ) ) ;
#17625=DIRECTION ( 'NONE',  ( 0.4472135954999587604, 0.7745966692414837373, 0.4472135954999567620 ) ) ;
#17626=VERTEX_POINT ( 'NONE', #3252 ) ;
#17633=EDGE_CURVE ( 'NONE', #16351, #13358, #2009, .T. ) ;
#17646=CARTESIAN_POINT ( 'NONE',  ( 2.775557561562891351E-14, 2.999999999999999112, -12.99999999999999822 ) ) ;
#17665=DIRECTION ( 'NONE',  ( -1.000000000000000000, 4.190823558986610327E-31, -1.733449886265890494E-32 ) ) ;
#17671=FACE_OUTER_BOUND ( 'NONE', #16863, .T. ) ;
#17697=AXIS2_PLACEMENT_3D ( 'NONE', #6799, #17259, #3042 ) ;
#17704=CARTESIAN_POINT ( 'NONE',  ( 37.52451905283849953, 10.90849364905388441, -10.18301270189226315 ) ) ;
#17722=CARTESIAN_POINT ( 'NONE',  ( 42.00000000000014921, 5.500000000000001776, 2.500000000000030198 ) ) ;
#17742=DIRECTION ( 'NONE',  ( -0.8660254037844395958, 0.4999999999999985567, 0.000000000000000000 ) ) ;
#17747=ORIENTED_EDGE ( 'NONE', *, *, #1455, .T. ) ;
#17748=EDGE_CURVE ( 'NONE', #15946, #23148, #4270, .T. ) ;
#17757=CARTESIAN_POINT ( 'NONE',  ( 2.775557561562891351E-14, 0.2500000000000002220, -6.499999999999950262 ) ) ;
#17769=CARTESIAN_POINT ( 'NONE',  ( 37.86602540378461157, 11.00000000000000000, -2.133974596215532316 ) ) ;
#17792=CIRCLE ( 'NONE', #22290, 0.5000000000000022204 ) ;
#17804=PLANE ( 'NONE',  #20448 ) ;
#17805=LINE ( 'NONE', #19685, #5733 ) ;
#17807=LINE ( 'NONE', #10737, #290 ) ;
#17820=ORIENTED_EDGE ( 'NONE', *, *, #21096, .T. ) ;
#17832=CARTESIAN_POINT ( 'NONE',  ( 42.00000000000012079, 0.000000000000000000, -12.49999999999999645 ) ) ;
#17848=EDGE_LOOP ( 'NONE', ( #895, #4820, #17221, #6877 ) ) ;
#17864=DIRECTION ( 'NONE',  ( 1.000000000000000000, -4.437342591868175641E-31, 3.330669073875457788E-16 ) ) ;
#17866=CARTESIAN_POINT ( 'NONE',  ( 37.00000000000011369, 11.00000000000000000, -10.00000000000000888 ) ) ;
#17867=EDGE_CURVE ( 'NONE', #18765, #5339, #2406, .T. ) ;
#17887=CARTESIAN_POINT ( 'NONE',  ( 37.00000000000014211, 10.75000000000000000, -2.566987298107808790 ) ) ;
#17889=EDGE_CURVE ( 'NONE', #17191, #15879, #4623, .T. ) ;
#17890=DIRECTION ( 'NONE',  ( -1.756300210255732376E-61, 4.190823558986625216E-31, 1.000000000000000000 ) ) ;
#17907=DIRECTION ( 'NONE',  ( 3.512600420511457844E-61, -4.190823558986624340E-31, -1.000000000000000000 ) ) ;
#17935=ORIENTED_EDGE ( 'NONE', *, *, #18576, .F. ) ;
#17972=CARTESIAN_POINT ( 'NONE',  ( 37.18301270189238039, 0.09150635094611105080, -10.52451905283837519 ) ) ;
#17980=CARTESIAN_POINT ( 'NONE',  ( 37.45482484129324519, 10.78777973366406329, -10.04362427881554964 ) ) ;
#17985=CARTESIAN_POINT ( 'NONE',  ( 5.551115123125782702E-14, 0.2500000000000002220, -2.566987298107781257 ) ) ;
#17995=VERTEX_POINT ( 'NONE', #10268 ) ;
#18001=DIRECTION ( 'NONE',  ( 0.000000000000000000, 0.000000000000000000, 1.000000000000000000 ) ) ;
#18005=DIRECTION ( 'NONE',  ( -4.190823558986625216E-31, 1.000000000000000000, -4.190823558986625216E-31 ) ) ;
#18008=CARTESIAN_POINT ( 'NONE',  ( 37.86602540378461157, 11.00000000000000000, -2.133974596215532316 ) ) ;
#18014=VECTOR ( 'NONE', #11713, 1000.000000000000000 ) ;
#18017=EDGE_LOOP ( 'NONE', ( #13977, #10278, #6062 ) ) ;
#18026=EDGE_CURVE ( 'NONE', #17226, #2694, #19437, .T. ) ;
#18071=CARTESIAN_POINT ( 'NONE',  ( 37.69139372032810797, 10.99999999999995914, -2.221290437944332119 ) ) ;
#18075=VERTEX_POINT ( 'NONE', #12731 ) ;
#18114=DIRECTION ( 'NONE',  ( -1.733449886265890494E-32, 7.264582621685753859E-63, 1.000000000000000000 ) ) ;
#18132=CARTESIAN_POINT ( 'NONE',  ( 37.48161866288226207, 0.1772999597157617346, -2.902788078020140272 ) ) ;
#18135=AXIS2_PLACEMENT_3D ( 'NONE', #21459, #19559, #8861 ) ;
#18139=ADVANCED_FACE ( 'NONE', ( #9082 ), #21684, .T. ) ;
#18144=CARTESIAN_POINT ( 'NONE',  ( 42.00000000000020606, 8.000000000000003553, -15.50000000000004086 ) ) ;
#18149=CIRCLE ( 'NONE', #5378, 0.5000000000000017764 ) ;
#18151=ADVANCED_FACE ( 'NONE', ( #12377 ), #17804, .T. ) ;
#18153=EDGE_CURVE ( 'NONE', #15246, #3085, #3568, .T. ) ;
#18157=ORIENTED_EDGE ( 'NONE', *, *, #8881, .T. ) ;
#18170=EDGE_CURVE ( 'NONE', #7709, #8906, #14795, .T. ) ;
#18191=CARTESIAN_POINT ( 'NONE',  ( 37.04362427881598308, 10.78777973366386078, -2.545175158707025265 ) ) ;
#18209=EDGE_CURVE ( 'NONE', #23148, #9224, #6506, .T. ) ;
#18216=CIRCLE ( 'NONE', #12182, 0.5000000000000022204 ) ;
#18220=ORIENTED_EDGE ( 'NONE', *, *, #13783, .F. ) ;
#18238=CARTESIAN_POINT ( 'NONE',  ( 37.86602540378459025, -1.387778780781445676E-14, -2.133974596215476360 ) ) ;
#18249=CARTESIAN_POINT ( 'NONE',  ( 37.60054931026179759, 0.05202134937413122051, -2.399450689738933384 ) ) ;
#18281=EDGE_CURVE ( 'NONE', #7570, #15190, #22665, .T. ) ;
#18287=DIRECTION ( 'NONE',  ( 1.000000000000000000, -4.190823558986610327E-31, 1.733449886265890494E-32 ) ) ;
#18291=CARTESIAN_POINT ( 'NONE',  ( 37.77870956205639885, 11.00000000000000000, -2.308606279672897887 ) ) ;
#18307=FACE_OUTER_BOUND ( 'NONE', #16142, .T. ) ;
#18345=CARTESIAN_POINT ( 'NONE',  ( 2.775557561562891351E-14, 10.75000000000000000, -10.43301270189220276 ) ) ;
#18368=CARTESIAN_POINT ( 'NONE',  ( 37.43301270189237329, 0.2499999999999700795, -2.999999999999904077 ) ) ;
#18375=VECTOR ( 'NONE', #21495, 1000.000000000000000 ) ;
#18392=ORIENTED_EDGE ( 'NONE', *, *, #20056, .F. ) ;
#18394=EDGE_LOOP ( 'NONE', ( #34, #5926, #22852, #17747 ) ) ;
#18401=PRODUCT_DEFINITION ( 'UNKNOWN', '', #14638, #11918 ) ;
#18408=CARTESIAN_POINT ( 'NONE',  ( 37.45482484129320255, 10.78777973366397092, -2.956375721184426819 ) ) ;
#18413=ORIENTED_EDGE ( 'NONE', *, *, #19893, .F. ) ;
#18420=DIRECTION ( 'NONE',  ( -1.000000000000000000, 4.190823558986610327E-31, -1.733449886265890494E-32 ) ) ;
#18438=ADVANCED_FACE ( 'NONE', ( #8835 ), #12503, .F. ) ;
#18463=EDGE_CURVE ( 'NONE', #22005, #12160, #13699, .T. ) ;
#18472=DIRECTION ( 'NONE',  ( 1.733449886265890494E-32, 4.190823558986611203E-31, -1.000000000000000000 ) ) ;
#18481=AXIS2_PLACEMENT_3D ( 'NONE', #16018, #264, #9084 ) ;
#18493=ORIENTED_EDGE ( 'NONE', *, *, #370, .F. ) ;
#18501=CARTESIAN_POINT ( 'NONE',  ( 2.775557561562891351E-14, 10.49999999999999822, -6.499999999999950262 ) ) ;
#18502=EDGE_LOOP ( 'NONE', ( #13677, #10931, #8963, #4189 ) ) ;
#18510=CARTESIAN_POINT ( 'NONE',  ( 37.43301270189233776, 10.75000000000000000, -9.999999999999994671 ) ) ;
#18541=AXIS2_PLACEMENT_3D ( 'NONE', #18930, #16908, #1476 ) ;
#18552=DIRECTION ( 'NONE',  ( -4.190823558986626092E-31, 1.000000000000000000, 4.190823558986610327E-31 ) ) ;
#18575=PLANE ( 'NONE',  #22226 ) ;
#18576=EDGE_CURVE ( 'NONE', #6390, #15040, #4103, .T. ) ;
#18583=LINE ( 'NONE', #13174, #21743 ) ;
#18585=CARTESIAN_POINT ( 'NONE',  ( 37.50000000000012790, -1.677151478558897161E-14, -2.316987298107702209 ) ) ;
#18588=ADVANCED_FACE ( 'NONE', ( #14584 ), #22111, .T. ) ;
#18607=CARTESIAN_POINT ( 'NONE',  ( 2.775557561562891351E-14, 0.5000000000000004441, -6.499999999999950262 ) ) ;
#18612=DIRECTION ( 'NONE',  ( 1.000000000000000000, -4.190823558986610327E-31, 1.733449886265890494E-32 ) ) ;
#18665=CARTESIAN_POINT ( 'NONE',  ( 2.775557561562891351E-14, 0.000000000000000000, -3.000000000000002665 ) ) ;
#18679=DIRECTION ( 'NONE',  ( 4.190823558986625216E-31, -1.000000000000000000, 4.190823558986625216E-31 ) ) ;
#18705=AXIS2_PLACEMENT_3D ( 'NONE', #10384, #8743, #6995 ) ;
#18706=DIRECTION ( 'NONE',  ( 1.733449886265891589E-32, -4.190823558986610327E-31, 1.000000000000000000 ) ) ;
#18723=CARTESIAN_POINT ( 'NONE',  ( 42.00000000000017764, 2.999999999999999112, 2.000000000000057288 ) ) ;
#18765=VERTEX_POINT ( 'NONE', #11972 ) ;
#18775=ORIENTED_EDGE ( 'NONE', *, *, #7690, .F. ) ;
#18799=FACE_OUTER_BOUND ( 'NONE', #17327, .T. ) ;
#18805=EDGE_CURVE ( 'NONE', #3237, #8906, #17792, .T. ) ;
#18808=DIRECTION ( 'NONE',  ( 4.190823558986626092E-31, -1.000000000000000000, -4.190823558986610327E-31 ) ) ;
#18816=AXIS2_PLACEMENT_3D ( 'NONE', #12218, #19405, #15863 ) ;
#18820=EDGE_LOOP ( 'NONE', ( #7540, #9851, #3861, #6034 ) ) ;
#18837=LINE ( 'NONE', #2843, #5580 ) ;
#18871=VERTEX_POINT ( 'NONE', #8686 ) ;
#18882=CIRCLE ( 'NONE', #478, 0.5000000000000004441 ) ;
#18890=ORIENTED_EDGE ( 'NONE', *, *, #21313, .T. ) ;
#18894=DIRECTION ( 'NONE',  ( 1.733449886265891589E-32, -4.190823558986610327E-31, 1.000000000000000000 ) ) ;
#18920=CARTESIAN_POINT ( 'NONE',  ( 2.775557561562891351E-14, 7.999999999999983125, 2.500000000000057732 ) ) ;
#18925=TOROIDAL_SURFACE ( 'NONE', #13667, 2.500000000000000000, 0.5000000000000000000 ) ;
#18930=CARTESIAN_POINT ( 'NONE',  ( 2.775557561562891351E-14, 10.75000000000000000, -6.499999999999950262 ) ) ;
#18932=FACE_OUTER_BOUND ( 'NONE', #9304, .T. ) ;
#18946=DIRECTION ( 'NONE',  ( 1.000000000000000000, 0.000000000000000000, 0.000000000000000000 ) ) ;
#18955=CARTESIAN_POINT ( 'NONE',  ( 42.50000000000020606, 2.999999999999999112, -13.00000000000002487 ) ) ;
#18960=DIRECTION ( 'NONE',  ( -1.000000000000000000, 4.190823558986610327E-31, -1.733449886265890494E-32 ) ) ;
#18975=ORIENTED_EDGE ( 'NONE', *, *, #6196, .T. ) ;
#18976=DIRECTION ( 'NONE',  ( -1.733449886265890494E-32, 7.264582621685754939E-63, 1.000000000000000000 ) ) ;
#18979=( BOUNDED_CURVE ( )  B_SPLINE_CURVE ( 3, ( #9465, #20644, #4512, #11677 ),
 .UNSPECIFIED., .F., .F. ) 
 B_SPLINE_CURVE_WITH_KNOTS ( ( 4, 4 ),
 ( 1.570796326794896558, 2.617993877991540597 ),
 .UNSPECIFIED. ) 
 CURVE ( )  GEOMETRIC_REPRESENTATION_ITEM ( )  RATIONAL_B_SPLINE_CURVE ( ( 1.000000000000000000, 0.9106836025229513298, 0.9106836025229513298, 1.000000000000000000 ) ) 
 REPRESENTATION_ITEM ( '' )  );
#19022=CARTESIAN_POINT ( 'NONE',  ( 37.46001462128849369, 0.1698019261547604186, -10.46001462128817927 ) ) ;
#19025=( NAMED_UNIT ( * ) SI_UNIT ( $, .STERADIAN. ) SOLID_ANGLE_UNIT ( ) );
#19033=DIRECTION ( 'NONE',  ( -1.000000000000000000, 1.492474417944849379E-16, 3.760416335592108037E-33 ) ) ;
#19034=CARTESIAN_POINT ( 'NONE',  ( 2.775557561562891351E-14, 0.000000000000000000, -6.499999999999950262 ) ) ;
#19035=ORIENTED_EDGE ( 'NONE', *, *, #18209, .T. ) ;
#19047=CARTESIAN_POINT ( 'NONE',  ( 2.775557561562891351E-14, 2.499999999999995115, -12.50000000000001066 ) ) ;
#19056=ORIENTED_EDGE ( 'NONE', *, *, #6635, .T. ) ;
#19067=TOROIDAL_SURFACE ( 'NONE', #22838, 2.500000000000000000, 0.5000000000000000000 ) ;
#19073=AXIS2_PLACEMENT_3D ( 'NONE', #12696, #10700, #21654 ) ;
#19098=CARTESIAN_POINT ( 'NONE',  ( 37.00000000000014211, 11.00000000000000000, -3.000000000000002665 ) ) ;
#19108=ORIENTED_EDGE ( 'NONE', *, *, #55, .T. ) ;
#19116=DIRECTION ( 'NONE',  ( 1.733449886265890494E-32, 4.190823558986611203E-31, -1.000000000000000000 ) ) ;
#19170=ORIENTED_EDGE ( 'NONE', *, *, #5382, .F. ) ;
#19205=CARTESIAN_POINT ( 'NONE',  ( 2.775557561562891351E-14, 11.00000000000000000, -6.499999999999950262 ) ) ;
#19228=ORIENTED_EDGE ( 'NONE', *, *, #18805, .T. ) ;
#19246=AXIS2_PLACEMENT_3D ( 'NONE', #19962, #6074, #14660 ) ;
#19250=ORIENTED_EDGE ( 'NONE', *, *, #15588, .T. ) ;
#19281=ADVANCED_FACE ( 'NONE', ( #3598 ), #10292, .F. ) ;
#19286=EDGE_LOOP ( 'NONE', ( #4860, #19542, #663, #4645 ) ) ;
#19293=CARTESIAN_POINT ( 'NONE',  ( 42.50000000000020606, 8.500000000000003553, -13.00000000000002487 ) ) ;
#19303=ADVANCED_FACE ( 'NONE', ( #7022 ), #12050, .F. ) ;
#19305=CARTESIAN_POINT ( 'NONE',  ( 2.775557561562891351E-14, 2.499999999999995115, -12.50000000000001066 ) ) ;
#19320=DIRECTION ( 'NONE',  ( 4.190823558986625216E-31, -1.000000000000000000, 4.190823558986625216E-31 ) ) ;
#19342=ORIENTED_EDGE ( 'NONE', *, *, #3481, .T. ) ;
#19352=PLANE ( 'NONE',  #10610 ) ;
#19364=VECTOR ( 'NONE', #3059, 1000.000000000000000 ) ;
#19373=DIRECTION ( 'NONE',  ( -4.190823558986625216E-31, 1.000000000000000000, -4.190823558986625216E-31 ) ) ;
#19405=DIRECTION ( 'NONE',  ( 1.733449886265891589E-32, -4.190823558986610327E-31, 1.000000000000000000 ) ) ;
#19408=CARTESIAN_POINT ( 'NONE',  ( 37.50000000000016342, 11.00000000000000355, -2.316987298107758164 ) ) ;
#19421=VECTOR ( 'NONE', #16700, 1000.000000000000000 ) ;
#19424=ORIENTED_EDGE ( 'NONE', *, *, #16971, .T. ) ;
#19430=CYLINDRICAL_SURFACE ( 'NONE', #9777, 0.5000000000000022204 ) ;
#19437=LINE ( 'NONE', #2020, #906 ) ;
#19454=ORIENTED_EDGE ( 'NONE', *, *, #15455, .T. ) ;
#19463=ADVANCED_FACE ( 'NONE', ( #15060, #16324 ), #9928, .F. ) ;
#19464=VECTOR ( 'NONE', #22112, 1000.000000000000000 ) ;
#19479=DIRECTION ( 'NONE',  ( 1.000000000000000000, -4.190823558986610327E-31, 1.733449886265890494E-32 ) ) ;
#19483=CIRCLE ( 'NONE', #16458, 0.5000000000000022204 ) ;
#19493=CARTESIAN_POINT ( 'NONE',  ( 42.00000000000012079, 0.5000000000000004441, -12.49999999999999645 ) ) ;
#19506=CARTESIAN_POINT ( 'NONE',  ( 37.35148779274808817, 10.63811079452496422, -10.35148779274853936 ) ) ;
#19542=ORIENTED_EDGE ( 'NONE', *, *, #4338, .T. ) ;
#19553=DIRECTION ( 'NONE',  ( 0.000000000000000000, 0.000000000000000000, 1.000000000000000000 ) ) ;
#19559=DIRECTION ( 'NONE',  ( 1.000000000000000000, -4.437342591868175641E-31, 3.330669073875457788E-16 ) ) ;
#19570=EDGE_CURVE ( 'NONE', #4397, #20741, #9934, .T. ) ;
#19590=DIRECTION ( 'NONE',  ( 0.000000000000000000, 0.000000000000000000, 1.000000000000000000 ) ) ;
#19628=ORIENTED_EDGE ( 'NONE', *, *, #3924, .F. ) ;
#19636=AXIS2_PLACEMENT_3D ( 'NONE', #17230, #905, #10176 ) ;
#19684=DIRECTION ( 'NONE',  ( -1.000000000000000000, 4.190823558986610327E-31, -1.733449886265890494E-32 ) ) ;
#19685=CARTESIAN_POINT ( 'NONE',  ( 2.775557561562891351E-14, 0.000000000000000000, -0.4999999999999865663 ) ) ;
#19695=VERTEX_POINT ( 'NONE', #2016 ) ;
#19710=AXIS2_PLACEMENT_3D ( 'NONE', #21097, #6739, #10379 ) ;
#19712=VECTOR ( 'NONE', #20631, 1000.000000000000000 ) ;
#19725=EDGE_CURVE ( 'NONE', #3408, #22005, #6933, .T. ) ;
#19745=CARTESIAN_POINT ( 'NONE',  ( 37.36637401601598185, 10.68627026436967675, -10.36637401601569231 ) ) ;
#19753=ORIENTED_EDGE ( 'NONE', *, *, #20349, .F. ) ;
#19767=DIRECTION ( 'NONE',  ( 1.000000000000000000, -4.437342591868175641E-31, 3.330669073875457788E-16 ) ) ;
#19810=ORIENTED_EDGE ( 'NONE', *, *, #18170, .F. ) ;
#19833=LINE ( 'NONE', #15818, #18375 ) ;
#19839=ORIENTED_EDGE ( 'NONE', *, *, #19941, .F. ) ;
#19845=CIRCLE ( 'NONE', #9706, 0.5000000000000017764 ) ;
#19846=CARTESIAN_POINT ( 'NONE',  ( 37.50000000000016342, -2.613291509943991698E-15, -10.68301270189226848 ) ) ;
#19893=EDGE_CURVE ( 'NONE', #23148, #17301, #13888, .T. ) ;
#19927=UNCERTAINTY_MEASURE_WITH_UNIT (LENGTH_MEASURE( 1.000000000000000082E-05 ), #16888, 'distance_accuracy_value', 'NONE');
#19941=EDGE_CURVE ( 'NONE', #12862, #1669, #22485, .T. ) ;
#19962=CARTESIAN_POINT ( 'NONE',  ( 2.775557561562891351E-14, 0.5000000000000004441, -2.133974596215532316 ) ) ;
#19967=CARTESIAN_POINT ( 'NONE',  ( 37.86602540378474657, 11.00000000000000533, -10.86602540378446591 ) ) ;
#19971=EDGE_CURVE ( 'NONE', #4498, #15879, #5790, .T. ) ;
#19979=CARTESIAN_POINT ( 'NONE',  ( 37.00000000000014211, 11.00000000000000000, -3.000000000000002665 ) ) ;
#19994=CARTESIAN_POINT ( 'NONE',  ( 37.86602540378461157, 11.00000000000000000, -6.500000000000005329 ) ) ;
#20008=AXIS2_PLACEMENT_3D ( 'NONE', #11724, #19033, #16773 ) ;
#20024=DIRECTION ( 'NONE',  ( 0.000000000000000000, 0.000000000000000000, 1.000000000000000000 ) ) ;
#20046=DIRECTION ( 'NONE',  ( 4.190823558986625216E-31, -1.000000000000000000, 4.190823558986625216E-31 ) ) ;
#20056=EDGE_CURVE ( 'NONE', #17226, #7345, #18216, .T. ) ;
#20057=CYLINDRICAL_SURFACE ( 'NONE', #3488, 0.5000000000000017764 ) ;
#20062=AXIS2_PLACEMENT_3D ( 'NONE', #21379, #3378, #19479 ) ;
#20066=VECTOR ( 'NONE', #5142, 1000.000000000000000 ) ;
#20067=ORIENTED_EDGE ( 'NONE', *, *, #17633, .F. ) ;
#20072=ORIENTED_EDGE ( 'NONE', *, *, #14558, .T. ) ;
#20080=AXIS2_PLACEMENT_3D ( 'NONE', #18607, #14841, #9435 ) ;
#20101=CARTESIAN_POINT ( 'NONE',  ( 0.000000000000000000, 1.387778780781445676E-14, -10.86602540378443749 ) ) ;
#20106=AXIS2_PLACEMENT_3D ( 'NONE', #17757, #1646, #8473 ) ;
#20114=CARTESIAN_POINT ( 'NONE',  ( 2.775557561562891351E-14, 10.99999999999998579, -0.4999999999999865663 ) ) ;
#20167=CARTESIAN_POINT ( 'NONE',  ( 37.43301270189239460, 10.75000000000000000, -6.500000000000019540 ) ) ;
#20183=ORIENTED_EDGE ( 'NONE', *, *, #1071, .T. ) ;
#20198=DIRECTION ( 'NONE',  ( 1.000000000000000000, -4.190823558986610327E-31, 1.733449886265890494E-32 ) ) ;
#20200=CARTESIAN_POINT ( 'NONE',  ( 37.86602540378461157, 0.000000000000000000, -10.86602540378449255 ) ) ;
#20241=SURFACE_STYLE_USAGE ( .BOTH. , #4212 ) ;
#20275=ORIENTED_EDGE ( 'NONE', *, *, #9390, .F. ) ;
#20278=ORIENTED_EDGE ( 'NONE', *, *, #12130, .F. ) ;
#20287=DIRECTION ( 'NONE',  ( 1.000000000000000000, 0.000000000000000000, 0.000000000000000000 ) ) ;
#20321=FACE_OUTER_BOUND ( 'NONE', #18017, .T. ) ;
#20323=DIRECTION ( 'NONE',  ( 1.733449886265891589E-32, -4.190823558986610327E-31, 1.000000000000000000 ) ) ;
#20326=ADVANCED_FACE ( 'NONE', ( #10204 ), #1287, .T. ) ;
#20347=FILL_AREA_STYLE_COLOUR ( '', #9619 ) ;
#20349=EDGE_CURVE ( 'NONE', #5046, #12160, #15155, .T. ) ;
#20353=ORIENTED_EDGE ( 'NONE', *, *, #3219, .T. ) ;
#20368=FACE_OUTER_BOUND ( 'NONE', #10537, .T. ) ;
#20417=AXIS2_PLACEMENT_3D ( 'NONE', #6105, #18679, #14805 ) ;
#20448=AXIS2_PLACEMENT_3D ( 'NONE', #3677, #12487, #19684 ) ;
#20455=DIRECTION ( 'NONE',  ( 1.733449886265891589E-32, -4.190823558986610327E-31, 1.000000000000000000 ) ) ;
#20471=EDGE_CURVE ( 'NONE', #14576, #7345, #13862, .T. ) ;
#20497=DIRECTION ( 'NONE',  ( 0.000000000000000000, 0.000000000000000000, -1.000000000000000000 ) ) ;
#20499=DIRECTION ( 'NONE',  ( -4.190823558986625216E-31, 1.000000000000000000, -4.190823558986625216E-31 ) ) ;
#20553=CARTESIAN_POINT ( 'NONE',  ( 37.60054931026106573, 0.05202134937407964371, -10.60054931026103553 ) ) ;
#20564=ORIENTED_EDGE ( 'NONE', *, *, #17748, .T. ) ;
#20580=CIRCLE ( 'NONE', #22459, 3.000000000000011546 ) ;
#20581=CARTESIAN_POINT ( 'NONE',  ( 37.00000000000011369, 11.00000000000000000, -10.00000000000000888 ) ) ;
#20605=AXIS2_PLACEMENT_3D ( 'NONE', #9907, #17060, #20618 ) ;
#20618=DIRECTION ( 'NONE',  ( 0.000000000000000000, 0.000000000000000000, 1.000000000000000000 ) ) ;
#20631=DIRECTION ( 'NONE',  ( 1.000000000000000000, -4.437342591868175641E-31, 3.330669073875457788E-16 ) ) ;
#20644=CARTESIAN_POINT ( 'NONE',  ( 37.68301270189235908, -1.703318040400119988E-14, -2.499999999999934275 ) ) ;
#20667=DIRECTION ( 'NONE',  ( 1.374679200952785197E-16, 1.000000000000000000, 0.000000000000000000 ) ) ;
#20681=CARTESIAN_POINT ( 'NONE',  ( 42.00000000000014921, 11.00000000000000000, -6.499999999999950262 ) ) ;
#20685=ORIENTED_EDGE ( 'NONE', *, *, #3646, .T. ) ;
#20702=DIRECTION ( 'NONE',  ( -1.000000000000000000, 4.190823558986610327E-31, -1.733449886265890494E-32 ) ) ;
#20729=LINE ( 'NONE', #19305, #2547 ) ;
#20736=AXIS2_PLACEMENT_3D ( 'NONE', #2365, #5802, #9318 ) ;
#20741=VERTEX_POINT ( 'NONE', #22780 ) ;
#20749=CARTESIAN_POINT ( 'NONE',  ( 2.775557561562891351E-14, 8.000000000000003553, -12.99999999999999822 ) ) ;
#20750=DIRECTION ( 'NONE',  ( 1.000000000000000000, -4.190823558986621713E-31, 0.000000000000000000 ) ) ;
#20789=CARTESIAN_POINT ( 'NONE',  ( 42.50000000000020606, 8.000000000000003553, -13.00000000000002487 ) ) ;
#20795=DIRECTION ( 'NONE',  ( 1.000000000000000000, -4.190823558986610327E-31, 1.733449886265890494E-32 ) ) ;
#20803=SURFACE_STYLE_USAGE ( .BOTH. , #22553 ) ;
#20811=FACE_OUTER_BOUND ( 'NONE', #2875, .T. ) ;
#20818=DIRECTION ( 'NONE',  ( 1.000000000000000000, -4.190823558986610327E-31, 1.733449886265890494E-32 ) ) ;
#20854=CARTESIAN_POINT ( 'NONE',  ( 2.775557561562891351E-14, 8.000000000000003553, -12.50000000000001066 ) ) ;
#20857=ORIENTED_EDGE ( 'NONE', *, *, #11239, .F. ) ;
#20859=ORIENTED_EDGE ( 'NONE', *, *, #11022, .F. ) ;
#20895=ADVANCED_FACE ( 'NONE', ( #2841 ), #13666, .F. ) ;
#20905=CARTESIAN_POINT ( 'NONE',  ( 37.29045043747289156, 0.08880391167994089452, -10.57823792062843715 ) ) ;
#20918=EDGE_LOOP ( 'NONE', ( #17935, #14101, #1154, #3088 ) ) ;
#20920=PLANE ( 'NONE',  #4658 ) ;
#20954=AXIS2_PLACEMENT_3D ( 'NONE', #4625, #1229, #16020 ) ;
#20971=ORIENTED_EDGE ( 'NONE', *, *, #11651, .F. ) ;
#20981=DIRECTION ( 'NONE',  ( 4.190823558986626092E-31, -1.000000000000000000, -4.190823558986610327E-31 ) ) ;
#21007=CARTESIAN_POINT ( 'NONE',  ( 5.551115123125782702E-14, 5.499999999999980460, 2.500000000000071498 ) ) ;
#21009=FACE_OUTER_BOUND ( 'NONE', #15419, .T. ) ;
#21020=VERTEX_POINT ( 'NONE', #5303 ) ;
#21035=ORIENTED_EDGE ( 'NONE', *, *, #9823, .T. ) ;
#21046=CYLINDRICAL_SURFACE ( 'NONE', #8191, 0.5000000000000022204 ) ;
#21088=CARTESIAN_POINT ( 'NONE',  ( 42.00000000000012079, 2.999999999999999112, -12.49999999999999645 ) ) ;
#21089=FACE_OUTER_BOUND ( 'NONE', #8726, .T. ) ;
#21090=MANIFOLD_SOLID_BREP ( 'Fillet3', #6565 ) ;
#21096=EDGE_CURVE ( 'NONE', #21020, #13739, #2807, .T. ) ;
#21097=CARTESIAN_POINT ( 'NONE',  ( 42.00000000000017764, 8.000000000000003553, 2.000000000000057288 ) ) ;
#21135=DIRECTION ( 'NONE',  ( 0.000000000000000000, 0.000000000000000000, 1.000000000000000000 ) ) ;
#21142=AXIS2_PLACEMENT_3D ( 'NONE', #9372, #12898, #7378 ) ;
#21156=DIRECTION ( 'NONE',  ( -3.330669073875457788E-16, -4.437342591868175641E-31, 1.000000000000000000 ) ) ;
#21192=DIRECTION ( 'NONE',  ( 3.330669073875457788E-16, 0.000000000000000000, -1.000000000000000000 ) ) ;
#21224=FACE_OUTER_BOUND ( 'NONE', #8450, .T. ) ;
#21235=LINE ( 'NONE', #22872, #5906 ) ;
#21242=ORIENTED_EDGE ( 'NONE', *, *, #17604, .F. ) ;
#21256=CARTESIAN_POINT ( 'NONE',  ( 42.00000000000014921, 10.49999999999999822, -6.499999999999950262 ) ) ;
#21288=( BOUNDED_CURVE ( )  B_SPLINE_CURVE ( 3, ( #23159, #19846, #17972, #16306 ),
 .UNSPECIFIED., .F., .F. ) 
 B_SPLINE_CURVE_WITH_KNOTS ( ( 4, 4 ),
 ( 1.570796326794896558, 2.617993877991513951 ),
 .UNSPECIFIED. ) 
 CURVE ( )  GEOMETRIC_REPRESENTATION_ITEM ( )  RATIONAL_B_SPLINE_CURVE ( ( 1.000000000000000000, 0.9106836025229557707, 0.9106836025229557707, 1.000000000000000000 ) ) 
 REPRESENTATION_ITEM ( '' )  );
#21293=EDGE_CURVE ( 'NONE', #21020, #12892, #12438, .T. ) ;
#21297=CARTESIAN_POINT ( 'NONE',  ( 2.775557561562891351E-14, 7.999999999999983125, 2.500000000000057732 ) ) ;
#21313=EDGE_CURVE ( 'NONE', #18075, #6443, #17124, .T. ) ;
#21336=CARTESIAN_POINT ( 'NONE',  ( 42.00000000000020606, 2.999999999999999112, -0.4999999999999449329 ) ) ;
#21378=DIRECTION ( 'NONE',  ( -4.190823558986625216E-31, 1.000000000000000000, -4.190823558986625216E-31 ) ) ;
#21379=CARTESIAN_POINT ( 'NONE',  ( 0.000000000000000000, 2.499999999999998668, 0.000000000000000000 ) ) ;
#21407=CARTESIAN_POINT ( 'NONE',  ( 37.43301270189239460, 10.75000000000000178, -10.00000000000007994 ) ) ;
#21425=ADVANCED_FACE ( 'NONE', ( #16423, #22085 ), #11139, .F. ) ;
#21434=CARTESIAN_POINT ( 'NONE',  ( 2.775557561562891351E-14, 2.999999999999992450, -0.4999999999999865663 ) ) ;
#21438=CIRCLE ( 'NONE', #8276, 3.000000000000011546 ) ;
#21445=ORIENTED_EDGE ( 'NONE', *, *, #5513, .T. ) ;
#21452=FACE_OUTER_BOUND ( 'NONE', #10435, .T. ) ;
#21459=CARTESIAN_POINT ( 'NONE',  ( 2.775557561562891351E-14, 11.00000000000000000, -9.999999999999968026 ) ) ;
#21460=ADVANCED_FACE ( 'NONE', ( #20321 ), #22038, .F. ) ;
#21495=DIRECTION ( 'NONE',  ( 1.733449886265891589E-32, -4.190823558986610327E-31, 1.000000000000000000 ) ) ;
#21503=AXIS2_PLACEMENT_3D ( 'NONE', #3216, #14262, #17543 ) ;
#21504=ORIENTED_EDGE ( 'NONE', *, *, #5936, .T. ) ;
#21505=EDGE_LOOP ( 'NONE', ( #8524, #17122, #9564, #17418, #7830, #12622, #16253, #7600 ) ) ;
#21526=ORIENTED_EDGE ( 'NONE', *, *, #5991, .T. ) ;
#21547=DIRECTION ( 'NONE',  ( 4.190823558986625216E-31, -1.000000000000000000, 4.190823558986625216E-31 ) ) ;
#21571=DIRECTION ( 'NONE',  ( 0.000000000000000000, 0.000000000000000000, 1.000000000000000000 ) ) ;
#21577=DIRECTION ( 'NONE',  ( 4.190823558986625216E-31, -1.000000000000000000, 4.190823558986625216E-31 ) ) ;
#21654=DIRECTION ( 'NONE',  ( 0.000000000000000000, 0.000000000000000000, 1.000000000000000000 ) ) ;
#21677=EDGE_CURVE ( 'NONE', #17626, #20741, #16751, .T. ) ;
#21684=CYLINDRICAL_SURFACE ( 'NONE', #10294, 3.000000000000011102 ) ;
#21687=CARTESIAN_POINT ( 'NONE',  ( 37.00000000000014211, 10.75000000000000000, -2.566987298107808790 ) ) ;
#21729=EDGE_LOOP ( 'NONE', ( #8899, #18493, #181, #5610 ) ) ;
#21741=FACE_OUTER_BOUND ( 'NONE', #3849, .T. ) ;
#21743=VECTOR ( 'NONE', #2108, 1000.000000000000000 ) ;
#21748=CARTESIAN_POINT ( 'NONE',  ( 37.54332536350041494, 0.1155932590976401775, -10.22062532321603712 ) ) ;
#21759=DIRECTION ( 'NONE',  ( -1.000000000000000000, 4.190823558986610327E-31, -1.733449886265890494E-32 ) ) ;
#21766=ADVANCED_FACE ( 'NONE', ( #3816 ), #13000, .F. ) ;
#21789=CARTESIAN_POINT ( 'NONE',  ( 37.69160037009711317, 0.02335407096321897094, -2.482824663591205461 ) ) ;
#21830=VECTOR ( 'NONE', #19767, 1000.000000000000000 ) ;
#21831=CARTESIAN_POINT ( 'NONE',  ( 37.34641016151397253, 10.60000000000007958, -2.653589838486262398 ) ) ;
#21852=DIRECTION ( 'NONE',  ( 1.733449886265891589E-32, -4.190823558986610327E-31, 1.000000000000000000 ) ) ;
#21857=AXIS2_PLACEMENT_3D ( 'NONE', #19979, #14909, #21861 ) ;
#21861=DIRECTION ( 'NONE',  ( 1.000000000000000000, 0.000000000000000000, 0.000000000000000000 ) ) ;
#21904=DIRECTION ( 'NONE',  ( 1.733449886265891589E-32, -4.190823558986610327E-31, 1.000000000000000000 ) ) ;
#21941=LINE ( 'NONE', #20167, #10517 ) ;
#21948=AXIS2_PLACEMENT_3D ( 'NONE', #23014, #10762, #10421 ) ;
#21950=CARTESIAN_POINT ( 'NONE',  ( 37.35148779274898345, 10.63811079452488961, -2.648512207251442874 ) ) ;
#21951=CIRCLE ( 'NONE', #17408, 0.5000000000000004441 ) ;
#21956=EDGE_CURVE ( 'NONE', #6443, #12862, #21235, .T. ) ;
#21965=DIRECTION ( 'NONE',  ( 3.330669073875454830E-16, 0.000000000000000000, -1.000000000000000000 ) ) ;
#21967=DIRECTION ( 'NONE',  ( -1.733449886265890494E-32, 7.264582621685753859E-63, 1.000000000000000000 ) ) ;
#22005=VERTEX_POINT ( 'NONE', #22756 ) ;
#22007=CARTESIAN_POINT ( 'NONE',  ( 37.42127086598689090, 0.2176602893534318184, -2.578729134013127755 ) ) ;
#22020=LINE ( 'NONE', #22252, #3303 ) ;
#22022=LINE ( 'NONE', #11305, #2541 ) ;
#22033=ORIENTED_EDGE ( 'NONE', *, *, #13569, .T. ) ;
#22038=( BOUNDED_SURFACE ( )  B_SPLINE_SURFACE ( 3, 2, ( 
 ( #9613, #7848, #22200 ),
 ( #1960, #10901, #9156 ),
 ( #16316, #221, #7388 ),
 ( #21748, #5630, #11598 ),
 ( #918, #19022, #20905 ),
 ( #13836, #20553, #13609 ),
 ( #10184, #2546, #6205 ),
 ( #13495, #13374, #17116 ) ),
 .UNSPECIFIED., .F., .F., .T. ) 
 B_SPLINE_SURFACE_WITH_KNOTS ( ( 4, 2, 2, 4 ),
 ( 3, 3 ),
 ( 3.665191429188095817, 3.926990816987244504, 4.188790204786393190, 4.712388980384689674 ),
 ( 0.000000000000000000, 1.000000000000000000 ),
 .UNSPECIFIED. ) 
 GEOMETRIC_REPRESENTATION_ITEM ( )  RATIONAL_B_SPLINE_SURFACE ( (
 ( 1.000000000000000000, 0.7905694150421765931, 1.000000000000000000),
 ( 1.000000000000000000, 0.8144940154005562150, 1.000000000000000000),
 ( 1.000000000000000000, 0.8408337562111960484, 1.000000000000000000),
 ( 1.000000000000000000, 0.8912170513578050457, 1.000000000000000000),
 ( 1.000000000000000000, 0.9152160911082583006, 1.000000000000000000),
 ( 1.000000000000000000, 0.9758108578640632969, 1.000000000000000000),
 ( 1.000000000000000000, 1.000509427570040133, 1.000000000000000000),
 ( 1.000000000000000000, 1.000000000000000000, 1.000000000000000000) ) ) 
 REPRESENTATION_ITEM ( '' )  SURFACE ( )  );
#22077=FACE_OUTER_BOUND ( 'NONE', #7154, .T. ) ;
#22085=FACE_BOUND ( 'NONE', #21505, .T. ) ;
#22111=CYLINDRICAL_SURFACE ( 'NONE', #1256, 3.000000000000011102 ) ;
#22112=DIRECTION ( 'NONE',  ( -1.733449886265891589E-32, 4.190823558986610327E-31, -1.000000000000000000 ) ) ;
#22113=PRESENTATION_STYLE_ASSIGNMENT (( #20241 ) ) ;
#22115=AXIS2_PLACEMENT_3D ( 'NONE', #4943, #2963, #5306 ) ;
#22131=AXIS2_PLACEMENT_3D ( 'NONE', #12639, #21378, #1481 ) ;
#22145=ORIENTED_EDGE ( 'NONE', *, *, #8507, .F. ) ;
#22147=ORIENTED_EDGE ( 'NONE', *, *, #19725, .T. ) ;
#22200=CARTESIAN_POINT ( 'NONE',  ( 37.00000000000030553, 0.2500000000000148215, -10.43301270189226138 ) ) ;
#22210=EDGE_CURVE ( 'NONE', #9224, #18765, #11655, .T. ) ;
#22226=AXIS2_PLACEMENT_3D ( 'NONE', #2681, #18808, #8101 ) ;
#22249=CARTESIAN_POINT ( 'NONE',  ( 2.775557561562891351E-14, 5.500000000000001776, -6.499999999999950262 ) ) ;
#22252=CARTESIAN_POINT ( 'NONE',  ( 42.00000000000014921, 0.000000000000000000, -6.499999999999950262 ) ) ;
#22261=UNCERTAINTY_MEASURE_WITH_UNIT (LENGTH_MEASURE( 1.000000000000000082E-05 ), #4666, 'distance_accuracy_value', 'NONE');
#22270=CARTESIAN_POINT ( 'NONE',  ( 2.775557561562891351E-14, 1.387778780781445676E-14, -9.999999999999968026 ) ) ;
#22290=AXIS2_PLACEMENT_3D ( 'NONE', #16911, #17864, #23167 ) ;
#22327=EDGE_CURVE ( 'NONE', #19695, #6443, #1630, .T. ) ;
#22337=PLANE ( 'NONE',  #11888 ) ;
#22347=DIRECTION ( 'NONE',  ( -1.000000000000000000, 4.190823558986610327E-31, -1.733449886265890494E-32 ) ) ;
#22353=EDGE_CURVE ( 'NONE', #4498, #16689, #13797, .T. ) ;
#22432=AXIS2_PLACEMENT_3D ( 'NONE', #20854, #18960, #17175 ) ;
#22451=DIRECTION ( 'NONE',  ( 0.000000000000000000, 0.000000000000000000, 1.000000000000000000 ) ) ;
#22459=AXIS2_PLACEMENT_3D ( 'NONE', #14956, #16711, #971 ) ;
#22462=CARTESIAN_POINT ( 'NONE',  ( 2.775557561562891351E-14, 2.999999999999999112, -15.49999999999998579 ) ) ;
#22483=ADVANCED_FACE ( 'NONE', ( #15015 ), #11144, .F. ) ;
#22485=LINE ( 'NONE', #4585, #23112 ) ;
#22541=EDGE_CURVE ( 'NONE', #15424, #7856, #15240, .T. ) ;
#22553=SURFACE_SIDE_STYLE ('',( #3145 ) ) ;
#22556=VERTEX_POINT ( 'NONE', #13841 ) ;
#22565=LINE ( 'NONE', #17367, #6637 ) ;
#22577=DIRECTION ( 'NONE',  ( 0.000000000000000000, 0.000000000000000000, -1.000000000000000000 ) ) ;
#22606=TOROIDAL_SURFACE ( 'NONE', #9088, 2.500000000000000000, 0.5000000000000000000 ) ;
#22632=SPHERICAL_SURFACE ( 'NONE', #20954, 0.5000000000000000000 ) ;
#22660=CARTESIAN_POINT ( 'NONE',  ( 42.50000000000014921, 8.000000000000003553, -14.99999999999998579 ) ) ;
#22665=CIRCLE ( 'NONE', #13643, 3.000000000000011102 ) ;
#22682=ORIENTED_EDGE ( 'NONE', *, *, #21956, .F. ) ;
#22690=FACE_OUTER_BOUND ( 'NONE', #9849, .T. ) ;
#22714=ORIENTED_EDGE ( 'NONE', *, *, #17604, .T. ) ;
#22748=VECTOR ( 'NONE', #13186, 1000.000000000000000 ) ;
#22756=CARTESIAN_POINT ( 'NONE',  ( 2.775557561562891351E-14, 2.499999999999998668, -0.4999999999999865663 ) ) ;
#22780=CARTESIAN_POINT ( 'NONE',  ( 42.50000000000014921, 8.000000000000003553, 2.000000000000071054 ) ) ;
#22795=FACE_BOUND ( 'NONE', #10597, .T. ) ;
#22834=CIRCLE ( 'NONE', #12679, 0.5000000000000004441 ) ;
#22838=AXIS2_PLACEMENT_3D ( 'NONE', #3650, #1656, #18114 ) ;
#22852=ORIENTED_EDGE ( 'NONE', *, *, #7340, .T. ) ;
#22872=CARTESIAN_POINT ( 'NONE',  ( 37.00000000000011369, 10.49999999999999822, -6.499999999999950262 ) ) ;
#22874=ORIENTED_EDGE ( 'NONE', *, *, #448, .T. ) ;
#22878=VERTEX_POINT ( 'NONE', #23115 ) ;
#22882=ORIENTED_EDGE ( 'NONE', *, *, #3219, .F. ) ;
#22983=CARTESIAN_POINT ( 'NONE',  ( 2.775557561562891351E-14, 10.99999999999998579, -2.133974596215532316 ) ) ;
#23003=CARTESIAN_POINT ( 'NONE',  ( 37.86602540378461157, 11.00000000000000000, -10.86602540378450676 ) ) ;
#23012=CARTESIAN_POINT ( 'NONE',  ( 37.68301270189238750, 11.00000000000000355, -10.50000000000005329 ) ) ;
#23014=CARTESIAN_POINT ( 'NONE',  ( 2.775557561562891351E-14, 11.00000000000000000, -6.499999999999950262 ) ) ;
#23016=ORIENTED_EDGE ( 'NONE', *, *, #16522, .T. ) ;
#23026=ORIENTED_EDGE ( 'NONE', *, *, #15455, .F. ) ;
#23034=DIRECTION ( 'NONE',  ( 0.000000000000000000, -1.000000000000000000, 2.168404344971006896E-16 ) ) ;
#23038=DIRECTION ( 'NONE',  ( 1.000000000000000000, 0.000000000000000000, 4.336808689942013792E-16 ) ) ;
#23056=EDGE_LOOP ( 'NONE', ( #15652, #12572, #2693 ) ) ;
#23063=EDGE_CURVE ( 'NONE', #13739, #16369, #22022, .T. ) ;
#23070=CARTESIAN_POINT ( 'NONE',  ( 2.775557561562891351E-14, 2.999999999999999112, -15.49999999999998579 ) ) ;
#23080=EDGE_CURVE ( 'NONE', #1098, #17626, #9328, .T. ) ;
#23094=ORIENTED_EDGE ( 'NONE', *, *, #11086, .F. ) ;
#23102=CYLINDRICAL_SURFACE ( 'NONE', #1361, 0.5000000000000004441 ) ;
#23109=DIRECTION ( 'NONE',  ( -1.000000000000000000, 4.190823558986610327E-31, -1.733449886265890494E-32 ) ) ;
#23110=ADVANCED_FACE ( 'NONE', ( #621 ), #9557, .T. ) ;
#23112=VECTOR ( 'NONE', #15987, 1000.000000000000000 ) ;
#23115=CARTESIAN_POINT ( 'NONE',  ( 37.00000000000014211, 0.5000000000000004441, -9.999999999999980460 ) ) ;
#23148=VERTEX_POINT ( 'NONE', #6029 ) ;
#23155=CARTESIAN_POINT ( 'NONE',  ( 0.000000000000000000, 2.499999999999998668, 0.000000000000000000 ) ) ;
#23159=CARTESIAN_POINT ( 'NONE',  ( 37.86602540378461157, 0.000000000000000000, -10.86602540378449255 ) ) ;
#23167=DIRECTION ( 'NONE',  ( 3.330669073875457788E-16, 0.000000000000000000, -1.000000000000000000 ) ) ;
#23182=EDGE_CURVE ( 'NONE', #22005, #14576, #18837, .T. ) ;
#23191=DIRECTION ( 'NONE',  ( 0.000000000000000000, 0.000000000000000000, 1.000000000000000000 ) ) ;
#23196=EDGE_CURVE ( 'NONE', #17995, #2357, #19845, .T. ) ;
#23201=VERTEX_POINT ( 'NONE', #13669 ) ;
#23249=DIRECTION ( 'NONE',  ( -1.000000000000000000, 4.190823558986610327E-31, -1.733449886265890494E-32 ) ) ;
ENDSEC;
END-ISO-10303-21;
